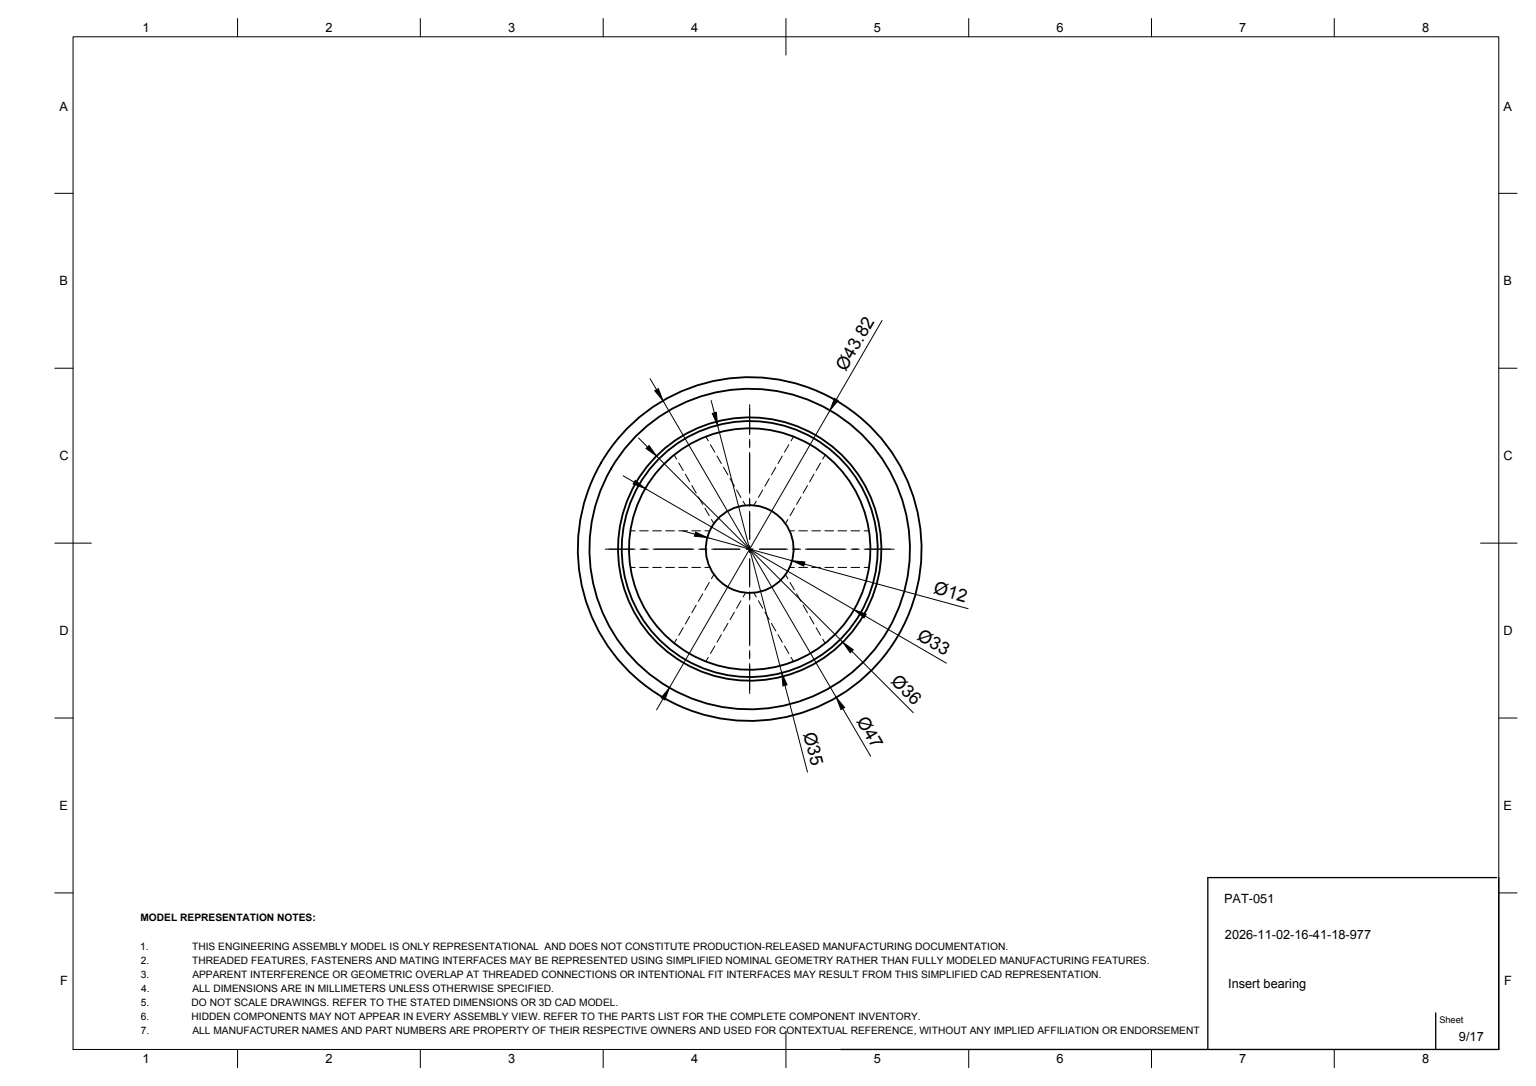
ISO-10303-21;
HEADER;
/* Generated by software containing ST-Developer
 * from STEP Tools, Inc. (www.steptools.com) 
 */

FILE_DESCRIPTION(
/* description */ ('Hand-crank flanged shaft unit'),
/* implementation_level */ '2;1');

FILE_NAME(
/* name */ 'Insert bearing.step',
/* time_stamp */ '2026-10-27T18:35:45-07:00',
/* author */ (''),
/* organization */ (''),
/* preprocessor_version */ 'ST-DEVELOPER v20.2',
/* originating_system */ 'Autodesk Translation Framework v15.17.0.0',
/* authorisation */ '');

FILE_SCHEMA (('AUTOMOTIVE_DESIGN { 1 0 10303 214 3 1 1 }'));
ENDSEC;

DATA;
#10=MECHANICAL_DESIGN_GEOMETRIC_PRESENTATION_REPRESENTATION('',(#289,#290),#6805);
#189=B_SPLINE_CURVE_WITH_KNOTS('',3,(#5317,#5318,#5319,#5320,#5321,#5322,
#5323,#5324,#5325,#5326),.UNSPECIFIED.,.F.,.F.,(4,2,2,2,4),(1.13193471301885,
1.22626174930539,1.32058878559194,1.41491753480854,1.50924628402513),
 .UNSPECIFIED.);
#190=B_SPLINE_CURVE_WITH_KNOTS('',3,(#5328,#5329,#5330,#5331,#5332,#5333,
#5334,#5335,#5336,#5337,#5338,#5339,#5340,#5341,#5342,#5343,#5344,#5345),
 .UNSPECIFIED.,.F.,.F.,(4,2,2,2,2,2,2,2,4),(0.377311571006283,0.471638607292829,
0.565965643579376,0.66029439279597,0.754623142012565,0.84895189122916,0.943280640445754,
1.0376076767323,1.13193471301885),.UNSPECIFIED.);
#191=B_SPLINE_CURVE_WITH_KNOTS('',3,(#5346,#5347,#5348,#5349,#5350,#5351,
#5352,#5353,#5354,#5355),.UNSPECIFIED.,.F.,.F.,(4,2,2,2,4),(1.50924628402513,
1.60357503324173,1.69790378245832,1.79223081874487,1.88655785503141),
 .UNSPECIFIED.);
#192=B_SPLINE_CURVE_WITH_KNOTS('',3,(#5358,#5359,#5360,#5361,#5362,#5363,
#5364,#5365,#5366,#5367,#5368,#5369,#5370,#5371,#5372,#5373,#5374,#5375,
#5376,#5377,#5378,#5379,#5380,#5381,#5382,#5383,#5384,#5385,#5386,#5387,
#5388,#5389,#5390,#5391),.UNSPECIFIED.,.T.,.F.,(4,2,2,2,2,2,2,2,2,2,2,2,
2,2,2,2,4),(0.,0.0955080856649705,0.191016171329941,0.286408845249646,0.38180151916935,
0.477194193089055,0.572586867008759,0.66809495267373,0.763603038338701,
0.859111124003671,0.954619209668642,1.05001188358835,1.14540455750805,1.24079723142776,
1.33618990534746,1.43169799101243,1.5272060766774),.UNSPECIFIED.);
#193=B_SPLINE_CURVE_WITH_KNOTS('',3,(#5394,#5395,#5396,#5397,#5398,#5399,
#5400,#5401,#5402,#5403,#5404,#5405,#5406,#5407,#5408,#5409,#5410,#5411,
#5412,#5413,#5414,#5415,#5416,#5417,#5418,#5419,#5420,#5421,#5422,#5423,
#5424,#5425,#5426,#5427),.UNSPECIFIED.,.T.,.F.,(4,2,2,2,2,2,2,2,2,2,2,2,
2,2,2,2,4),(0.,0.0955080856649706,0.191016171329941,0.286408845249646,0.381801519169351,
0.477194193089055,0.57258686700876,0.668094952673731,0.763603038338701,
0.859111124003672,0.954619209668642,1.05001188358835,1.14540455750805,1.24079723142776,
1.33618990534746,1.43169799101243,1.5272060766774),.UNSPECIFIED.);
#194=B_SPLINE_CURVE_WITH_KNOTS('',3,(#5431,#5432,#5433,#5434,#5435,#5436,
#5437,#5438,#5439,#5440),.UNSPECIFIED.,.F.,.F.,(4,2,2,2,4),(1.13193471301885,
1.22626174930539,1.32058878559194,1.41491753480854,1.50924628402513),
 .UNSPECIFIED.);
#195=B_SPLINE_CURVE_WITH_KNOTS('',3,(#5442,#5443,#5444,#5445,#5446,#5447,
#5448,#5449,#5450,#5451,#5452,#5453,#5454,#5455,#5456,#5457,#5458,#5459),
 .UNSPECIFIED.,.F.,.F.,(4,2,2,2,2,2,2,2,4),(0.377311571006283,0.47163860729283,
0.565965643579376,0.660294392795971,0.754623142012565,0.84895189122916,
0.943280640445755,1.0376076767323,1.13193471301885),.UNSPECIFIED.);
#196=B_SPLINE_CURVE_WITH_KNOTS('',3,(#5460,#5461,#5462,#5463,#5464,#5465,
#5466,#5467,#5468,#5469),.UNSPECIFIED.,.F.,.F.,(4,2,2,2,4),(1.50924628402513,
1.60357503324173,1.69790378245832,1.79223081874487,1.88655785503141),
 .UNSPECIFIED.);
#197=B_SPLINE_CURVE_WITH_KNOTS('',3,(#5478,#5479,#5480,#5481,#5482,#5483,
#5484,#5485,#5486,#5487,#5488,#5489,#5490,#5491,#5492,#5493,#5494,#5495),
 .UNSPECIFIED.,.F.,.F.,(4,2,2,2,2,2,2,2,4),(0.377311571006282,0.471638607292829,
0.565965643579376,0.660294392795971,0.754623142012565,0.84895189122916,
0.943280640445754,1.0376076767323,1.13193471301885),.UNSPECIFIED.);
#198=B_SPLINE_CURVE_WITH_KNOTS('',3,(#5497,#5498,#5499,#5500,#5501,#5502,
#5503,#5504,#5505,#5506),.UNSPECIFIED.,.F.,.F.,(4,2,2,2,4),(1.13193471301885,
1.22626174930539,1.32058878559194,1.41491753480854,1.50924628402513),
 .UNSPECIFIED.);
#199=B_SPLINE_CURVE_WITH_KNOTS('',3,(#5507,#5508,#5509,#5510,#5511,#5512,
#5513,#5514,#5515,#5516),.UNSPECIFIED.,.F.,.F.,(4,2,2,2,4),(1.50924628402513,
1.60357503324172,1.69790378245832,1.79223081874487,1.88655785503141),
 .UNSPECIFIED.);
#200=B_SPLINE_CURVE_WITH_KNOTS('',3,(#5519,#5520,#5521,#5522,#5523,#5524,
#5525,#5526,#5527,#5528,#5529,#5530,#5531,#5532,#5533,#5534,#5535,#5536),
 .UNSPECIFIED.,.F.,.F.,(4,2,2,2,2,2,2,2,4),(0.377311571006283,0.47163860729283,
0.565965643579376,0.660294392795971,0.754623142012565,0.84895189122916,
0.943280640445754,1.0376076767323,1.13193471301885),.UNSPECIFIED.);
#201=B_SPLINE_CURVE_WITH_KNOTS('',3,(#5538,#5539,#5540,#5541,#5542,#5543,
#5544,#5545,#5546,#5547),.UNSPECIFIED.,.F.,.F.,(4,2,2,2,4),(1.13193471301885,
1.22626174930539,1.32058878559194,1.41491753480854,1.50924628402513),
 .UNSPECIFIED.);
#202=B_SPLINE_CURVE_WITH_KNOTS('',3,(#5548,#5549,#5550,#5551,#5552,#5553,
#5554,#5555,#5556,#5557),.UNSPECIFIED.,.F.,.F.,(4,2,2,2,4),(1.50924628402513,
1.60357503324173,1.69790378245832,1.79223081874487,1.88655785503141),
 .UNSPECIFIED.);
#203=B_SPLINE_CURVE_WITH_KNOTS('',3,(#5560,#5561,#5562,#5563,#5564,#5565,
#5566,#5567,#5568,#5569,#5570,#5571,#5572,#5573,#5574,#5575,#5576,#5577),
 .UNSPECIFIED.,.F.,.F.,(4,2,2,2,2,2,2,2,4),(0.377311571006282,0.471638607292829,
0.565965643579376,0.66029439279597,0.754623142012565,0.84895189122916,0.943280640445754,
1.0376076767323,1.13193471301885),.UNSPECIFIED.);
#204=B_SPLINE_CURVE_WITH_KNOTS('',3,(#5579,#5580,#5581,#5582,#5583,#5584,
#5585,#5586,#5587,#5588),.UNSPECIFIED.,.F.,.F.,(4,2,2,2,4),(1.13193471301885,
1.22626174930539,1.32058878559194,1.41491753480854,1.50924628402513),
 .UNSPECIFIED.);
#205=B_SPLINE_CURVE_WITH_KNOTS('',3,(#5589,#5590,#5591,#5592,#5593,#5594,
#5595,#5596,#5597,#5598),.UNSPECIFIED.,.F.,.F.,(4,2,2,2,4),(1.50924628402513,
1.60357503324172,1.69790378245832,1.79223081874487,1.88655785503141),
 .UNSPECIFIED.);
#206=B_SPLINE_CURVE_WITH_KNOTS('',3,(#5601,#5602,#5603,#5604,#5605,#5606,
#5607,#5608,#5609,#5610,#5611,#5612,#5613,#5614,#5615,#5616,#5617,#5618),
 .UNSPECIFIED.,.F.,.F.,(4,2,2,2,2,2,2,2,4),(0.377311571006283,0.471638607292829,
0.565965643579376,0.660294392795971,0.754623142012565,0.84895189122916,
0.943280640445755,1.0376076767323,1.13193471301885),.UNSPECIFIED.);
#207=B_SPLINE_CURVE_WITH_KNOTS('',3,(#5620,#5621,#5622,#5623,#5624,#5625,
#5626,#5627,#5628,#5629),.UNSPECIFIED.,.F.,.F.,(4,2,2,2,4),(1.13193471301885,
1.22626174930539,1.32058878559194,1.41491753480854,1.50924628402513),
 .UNSPECIFIED.);
#208=B_SPLINE_CURVE_WITH_KNOTS('',3,(#5630,#5631,#5632,#5633,#5634,#5635,
#5636,#5637,#5638,#5639),.UNSPECIFIED.,.F.,.F.,(4,2,2,2,4),(1.50924628402513,
1.60357503324172,1.69790378245832,1.79223081874487,1.88655785503141),
 .UNSPECIFIED.);
#209=B_SPLINE_CURVE_WITH_KNOTS('',3,(#5643,#5644,#5645,#5646,#5647,#5648,
#5649,#5650,#5651,#5652,#5653,#5654,#5655,#5656,#5657,#5658,#5659,#5660,
#5661,#5662,#5663,#5664,#5665,#5666,#5667,#5668,#5669,#5670,#5671,#5672,
#5673,#5674,#5675,#5676),.UNSPECIFIED.,.T.,.F.,(4,2,2,2,2,2,2,2,2,2,2,2,
2,2,2,2,4),(0.,0.0955080856649705,0.191016171329941,0.286408845249646,0.38180151916935,
0.477194193089055,0.572586867008759,0.66809495267373,0.7636030383387,0.859111124003671,
0.954619209668642,1.05001188358835,1.14540455750805,1.24079723142776,1.33618990534746,
1.43169799101243,1.5272060766774),.UNSPECIFIED.);
#210=B_SPLINE_CURVE_WITH_KNOTS('',3,(#5679,#5680,#5681,#5682,#5683,#5684,
#5685,#5686,#5687,#5688,#5689,#5690,#5691,#5692,#5693,#5694,#5695,#5696,
#5697,#5698,#5699,#5700,#5701,#5702,#5703,#5704,#5705,#5706,#5707,#5708,
#5709,#5710,#5711,#5712),.UNSPECIFIED.,.T.,.F.,(4,2,2,2,2,2,2,2,2,2,2,2,
2,2,2,2,4),(0.,0.0955080856649706,0.191016171329941,0.286408845249646,0.381801519169351,
0.477194193089055,0.57258686700876,0.668094952673731,0.763603038338701,
0.859111124003672,0.954619209668642,1.05001188358835,1.14540455750805,1.24079723142776,
1.33618990534746,1.43169799101243,1.5272060766774),.UNSPECIFIED.);
#211=B_SPLINE_CURVE_WITH_KNOTS('',3,(#5717,#5718,#5719,#5720,#5721,#5722,
#5723,#5724,#5725,#5726,#5727,#5728,#5729,#5730,#5731,#5732,#5733,#5734,
#5735,#5736,#5737,#5738,#5739,#5740,#5741,#5742,#5743,#5744,#5745,#5746,
#5747,#5748,#5749,#5750),.UNSPECIFIED.,.T.,.F.,(4,2,2,2,2,2,2,2,2,2,2,2,
2,2,2,2,4),(0.,0.0955080856649705,0.191016171329941,0.286408845249646,0.38180151916935,
0.477194193089055,0.572586867008759,0.66809495267373,0.7636030383387,0.859111124003671,
0.954619209668642,1.05001188358835,1.14540455750805,1.24079723142776,1.33618990534746,
1.43169799101243,1.5272060766774),.UNSPECIFIED.);
#212=B_SPLINE_CURVE_WITH_KNOTS('',3,(#5753,#5754,#5755,#5756,#5757,#5758,
#5759,#5760,#5761,#5762,#5763,#5764,#5765,#5766,#5767,#5768,#5769,#5770,
#5771,#5772,#5773,#5774,#5775,#5776,#5777,#5778,#5779,#5780,#5781,#5782,
#5783,#5784,#5785,#5786),.UNSPECIFIED.,.T.,.F.,(4,2,2,2,2,2,2,2,2,2,2,2,
2,2,2,2,4),(0.,0.0955080856649706,0.191016171329941,0.286408845249646,0.381801519169351,
0.477194193089055,0.57258686700876,0.668094952673731,0.763603038338701,
0.859111124003672,0.954619209668642,1.05001188358835,1.14540455750805,1.24079723142776,
1.33618990534746,1.43169799101243,1.5272060766774),.UNSPECIFIED.);
#238=SPHERICAL_SURFACE('',#3719,2.35);
#249=SHAPE_REPRESENTATION_RELATIONSHIP('SRR','None',#6911,#269);
#269=ADVANCED_BREP_SHAPE_REPRESENTATION('',(#310,#311),#6794);
#289=STYLED_ITEM('',(#7091),#310);
#290=STYLED_ITEM('',(#7091),#311);
#310=MANIFOLD_SOLID_BREP('Body1',#3330);
#311=MANIFOLD_SOLID_BREP('Body2',#3331);
#372=FACE_BOUND('',#836,.T.);
#373=FACE_BOUND('',#838,.T.);
#374=FACE_BOUND('',#839,.T.);
#375=FACE_BOUND('',#841,.T.);
#376=FACE_BOUND('',#845,.T.);
#377=FACE_BOUND('',#846,.T.);
#378=FACE_BOUND('',#847,.T.);
#379=FACE_BOUND('',#848,.T.);
#380=FACE_BOUND('',#849,.T.);
#381=FACE_BOUND('',#850,.T.);
#382=FACE_BOUND('',#856,.T.);
#383=FACE_BOUND('',#858,.T.);
#384=FACE_BOUND('',#861,.T.);
#385=FACE_BOUND('',#863,.T.);
#386=FACE_BOUND('',#864,.T.);
#387=FACE_BOUND('',#865,.T.);
#388=FACE_BOUND('',#866,.T.);
#389=FACE_BOUND('',#867,.T.);
#390=FACE_BOUND('',#868,.T.);
#454=PLANE('',#3717);
#455=PLANE('',#3722);
#456=PLANE('',#3732);
#457=PLANE('',#3734);
#458=PLANE('',#3738);
#594=FACE_OUTER_BOUND('',#834,.T.);
#595=FACE_OUTER_BOUND('',#835,.T.);
#596=FACE_OUTER_BOUND('',#837,.T.);
#597=FACE_OUTER_BOUND('',#840,.T.);
#598=FACE_OUTER_BOUND('',#842,.T.);
#599=FACE_OUTER_BOUND('',#843,.T.);
#600=FACE_OUTER_BOUND('',#844,.T.);
#601=FACE_OUTER_BOUND('',#851,.T.);
#602=FACE_OUTER_BOUND('',#852,.T.);
#603=FACE_OUTER_BOUND('',#853,.T.);
#604=FACE_OUTER_BOUND('',#854,.T.);
#605=FACE_OUTER_BOUND('',#855,.T.);
#606=FACE_OUTER_BOUND('',#857,.T.);
#607=FACE_OUTER_BOUND('',#859,.T.);
#608=FACE_OUTER_BOUND('',#860,.T.);
#609=FACE_OUTER_BOUND('',#862,.T.);
#834=EDGE_LOOP('',(#2577,#2578,#2579,#2580));
#835=EDGE_LOOP('',(#2581));
#836=EDGE_LOOP('',(#2582));
#837=EDGE_LOOP('',(#2583,#2584));
#838=EDGE_LOOP('',(#2585));
#839=EDGE_LOOP('',(#2586));
#840=EDGE_LOOP('',(#2587));
#841=EDGE_LOOP('',(#2588));
#842=EDGE_LOOP('',(#2589,#2590,#2591,#2592,#2593,#2594));
#843=EDGE_LOOP('',(#2595,#2596,#2597,#2598,#2599,#2600));
#844=EDGE_LOOP('',(#2601,#2602,#2603,#2604));
#845=EDGE_LOOP('',(#2605,#2606,#2607));
#846=EDGE_LOOP('',(#2608,#2609,#2610));
#847=EDGE_LOOP('',(#2611,#2612,#2613));
#848=EDGE_LOOP('',(#2614,#2615,#2616));
#849=EDGE_LOOP('',(#2617,#2618,#2619));
#850=EDGE_LOOP('',(#2620,#2621,#2622));
#851=EDGE_LOOP('',(#2623,#2624,#2625,#2626,#2627,#2628));
#852=EDGE_LOOP('',(#2629,#2630,#2631,#2632,#2633,#2634));
#853=EDGE_LOOP('',(#2635,#2636,#2637,#2638,#2639,#2640));
#854=EDGE_LOOP('',(#2641,#2642,#2643,#2644,#2645,#2646));
#855=EDGE_LOOP('',(#2647));
#856=EDGE_LOOP('',(#2648));
#857=EDGE_LOOP('',(#2649));
#858=EDGE_LOOP('',(#2650));
#859=EDGE_LOOP('',(#2651,#2652,#2653,#2654));
#860=EDGE_LOOP('',(#2655));
#861=EDGE_LOOP('',(#2656));
#862=EDGE_LOOP('',(#2657,#2658,#2659,#2660));
#863=EDGE_LOOP('',(#2661));
#864=EDGE_LOOP('',(#2662));
#865=EDGE_LOOP('',(#2663));
#866=EDGE_LOOP('',(#2664));
#867=EDGE_LOOP('',(#2665));
#868=EDGE_LOOP('',(#2666));
#1075=LINE('',#5302,#1303);
#1076=LINE('',#5357,#1304);
#1077=LINE('',#5429,#1305);
#1078=LINE('',#5474,#1306);
#1079=LINE('',#5642,#1307);
#1080=LINE('',#5713,#1308);
#1081=LINE('',#5716,#1309);
#1082=LINE('',#5787,#1310);
#1083=LINE('',#5797,#1311);
#1084=LINE('',#5802,#1312);
#1303=VECTOR('',#4358,1.8);
#1304=VECTOR('',#4375,0.25);
#1305=VECTOR('',#4378,0.25);
#1306=VECTOR('',#4383,1.65);
#1307=VECTOR('',#4388,0.25);
#1308=VECTOR('',#4391,0.25);
#1309=VECTOR('',#4394,0.25);
#1310=VECTOR('',#4397,0.25);
#1311=VECTOR('',#4410,1.75);
#1312=VECTOR('',#4417,0.6);
#1506=CIRCLE('',#3715,1.8);
#1507=CIRCLE('',#3716,1.8);
#1508=CIRCLE('',#3718,2.19089023002066);
#1509=CIRCLE('',#3720,2.35);
#1510=CIRCLE('',#3721,2.19089023002066);
#1511=CIRCLE('',#3726,1.65);
#1512=CIRCLE('',#3727,1.65);
#1513=CIRCLE('',#3733,0.6);
#1514=CIRCLE('',#3735,1.75);
#1515=CIRCLE('',#3737,1.75);
#1516=CIRCLE('',#3739,0.6);
#1679=VERTEX_POINT('',#5299);
#1680=VERTEX_POINT('',#5301);
#1681=VERTEX_POINT('',#5305);
#1682=VERTEX_POINT('',#5308);
#1683=VERTEX_POINT('',#5309);
#1684=VERTEX_POINT('',#5311);
#1685=VERTEX_POINT('',#5315);
#1686=VERTEX_POINT('',#5316);
#1687=VERTEX_POINT('',#5327);
#1688=VERTEX_POINT('',#5356);
#1689=VERTEX_POINT('',#5393);
#1690=VERTEX_POINT('',#5428);
#1691=VERTEX_POINT('',#5430);
#1692=VERTEX_POINT('',#5441);
#1693=VERTEX_POINT('',#5471);
#1694=VERTEX_POINT('',#5473);
#1695=VERTEX_POINT('',#5476);
#1696=VERTEX_POINT('',#5477);
#1697=VERTEX_POINT('',#5496);
#1698=VERTEX_POINT('',#5517);
#1699=VERTEX_POINT('',#5518);
#1700=VERTEX_POINT('',#5537);
#1701=VERTEX_POINT('',#5558);
#1702=VERTEX_POINT('',#5559);
#1703=VERTEX_POINT('',#5578);
#1704=VERTEX_POINT('',#5599);
#1705=VERTEX_POINT('',#5600);
#1706=VERTEX_POINT('',#5619);
#1707=VERTEX_POINT('',#5641);
#1708=VERTEX_POINT('',#5678);
#1709=VERTEX_POINT('',#5715);
#1710=VERTEX_POINT('',#5752);
#1711=VERTEX_POINT('',#5789);
#1712=VERTEX_POINT('',#5792);
#1713=VERTEX_POINT('',#5795);
#1714=VERTEX_POINT('',#5799);
#2006=EDGE_CURVE('',#1679,#1679,#1506,.T.);
#2007=EDGE_CURVE('',#1679,#1680,#1075,.T.);
#2008=EDGE_CURVE('',#1680,#1680,#1507,.T.);
#2009=EDGE_CURVE('',#1681,#1681,#1508,.T.);
#2010=EDGE_CURVE('',#1682,#1683,#1509,.T.);
#2011=EDGE_CURVE('',#1684,#1684,#1510,.T.);
#2012=EDGE_CURVE('',#1685,#1686,#189,.T.);
#2013=EDGE_CURVE('',#1687,#1685,#190,.T.);
#2014=EDGE_CURVE('',#1686,#1687,#191,.T.);
#2015=EDGE_CURVE('',#1686,#1688,#1076,.T.);
#2016=EDGE_CURVE('',#1688,#1688,#192,.T.);
#2017=EDGE_CURVE('',#1689,#1689,#193,.T.);
#2018=EDGE_CURVE('',#1689,#1690,#1077,.T.);
#2019=EDGE_CURVE('',#1691,#1690,#194,.T.);
#2020=EDGE_CURVE('',#1692,#1691,#195,.T.);
#2021=EDGE_CURVE('',#1690,#1692,#196,.T.);
#2022=EDGE_CURVE('',#1693,#1693,#1511,.T.);
#2023=EDGE_CURVE('',#1693,#1694,#1078,.T.);
#2024=EDGE_CURVE('',#1694,#1694,#1512,.T.);
#2025=EDGE_CURVE('',#1695,#1696,#197,.T.);
#2026=EDGE_CURVE('',#1696,#1697,#198,.T.);
#2027=EDGE_CURVE('',#1697,#1695,#199,.T.);
#2028=EDGE_CURVE('',#1698,#1699,#200,.T.);
#2029=EDGE_CURVE('',#1699,#1700,#201,.T.);
#2030=EDGE_CURVE('',#1700,#1698,#202,.T.);
#2031=EDGE_CURVE('',#1701,#1702,#203,.T.);
#2032=EDGE_CURVE('',#1702,#1703,#204,.T.);
#2033=EDGE_CURVE('',#1703,#1701,#205,.T.);
#2034=EDGE_CURVE('',#1704,#1705,#206,.T.);
#2035=EDGE_CURVE('',#1705,#1706,#207,.T.);
#2036=EDGE_CURVE('',#1706,#1704,#208,.T.);
#2037=EDGE_CURVE('',#1697,#1707,#1079,.T.);
#2038=EDGE_CURVE('',#1707,#1707,#209,.T.);
#2039=EDGE_CURVE('',#1708,#1708,#210,.T.);
#2040=EDGE_CURVE('',#1708,#1700,#1080,.T.);
#2041=EDGE_CURVE('',#1703,#1709,#1081,.T.);
#2042=EDGE_CURVE('',#1709,#1709,#211,.T.);
#2043=EDGE_CURVE('',#1710,#1710,#212,.T.);
#2044=EDGE_CURVE('',#1710,#1706,#1082,.T.);
#2045=EDGE_CURVE('',#1711,#1711,#1513,.T.);
#2046=EDGE_CURVE('',#1712,#1712,#1514,.T.);
#2047=EDGE_CURVE('',#1713,#1713,#1515,.T.);
#2048=EDGE_CURVE('',#1713,#1712,#1083,.T.);
#2049=EDGE_CURVE('',#1714,#1714,#1516,.T.);
#2050=EDGE_CURVE('',#1714,#1711,#1084,.T.);
#2577=ORIENTED_EDGE('',*,*,#2006,.T.);
#2578=ORIENTED_EDGE('',*,*,#2007,.T.);
#2579=ORIENTED_EDGE('',*,*,#2008,.F.);
#2580=ORIENTED_EDGE('',*,*,#2007,.F.);
#2581=ORIENTED_EDGE('',*,*,#2009,.F.);
#2582=ORIENTED_EDGE('',*,*,#2008,.T.);
#2583=ORIENTED_EDGE('',*,*,#2010,.T.);
#2584=ORIENTED_EDGE('',*,*,#2010,.F.);
#2585=ORIENTED_EDGE('',*,*,#2009,.T.);
#2586=ORIENTED_EDGE('',*,*,#2011,.F.);
#2587=ORIENTED_EDGE('',*,*,#2011,.T.);
#2588=ORIENTED_EDGE('',*,*,#2006,.F.);
#2589=ORIENTED_EDGE('',*,*,#2012,.F.);
#2590=ORIENTED_EDGE('',*,*,#2013,.F.);
#2591=ORIENTED_EDGE('',*,*,#2014,.F.);
#2592=ORIENTED_EDGE('',*,*,#2015,.T.);
#2593=ORIENTED_EDGE('',*,*,#2016,.F.);
#2594=ORIENTED_EDGE('',*,*,#2015,.F.);
#2595=ORIENTED_EDGE('',*,*,#2017,.F.);
#2596=ORIENTED_EDGE('',*,*,#2018,.T.);
#2597=ORIENTED_EDGE('',*,*,#2019,.F.);
#2598=ORIENTED_EDGE('',*,*,#2020,.F.);
#2599=ORIENTED_EDGE('',*,*,#2021,.F.);
#2600=ORIENTED_EDGE('',*,*,#2018,.F.);
#2601=ORIENTED_EDGE('',*,*,#2022,.F.);
#2602=ORIENTED_EDGE('',*,*,#2023,.T.);
#2603=ORIENTED_EDGE('',*,*,#2024,.T.);
#2604=ORIENTED_EDGE('',*,*,#2023,.F.);
#2605=ORIENTED_EDGE('',*,*,#2013,.T.);
#2606=ORIENTED_EDGE('',*,*,#2012,.T.);
#2607=ORIENTED_EDGE('',*,*,#2014,.T.);
#2608=ORIENTED_EDGE('',*,*,#2020,.T.);
#2609=ORIENTED_EDGE('',*,*,#2019,.T.);
#2610=ORIENTED_EDGE('',*,*,#2021,.T.);
#2611=ORIENTED_EDGE('',*,*,#2025,.T.);
#2612=ORIENTED_EDGE('',*,*,#2026,.T.);
#2613=ORIENTED_EDGE('',*,*,#2027,.T.);
#2614=ORIENTED_EDGE('',*,*,#2028,.T.);
#2615=ORIENTED_EDGE('',*,*,#2029,.T.);
#2616=ORIENTED_EDGE('',*,*,#2030,.T.);
#2617=ORIENTED_EDGE('',*,*,#2031,.T.);
#2618=ORIENTED_EDGE('',*,*,#2032,.T.);
#2619=ORIENTED_EDGE('',*,*,#2033,.T.);
#2620=ORIENTED_EDGE('',*,*,#2034,.T.);
#2621=ORIENTED_EDGE('',*,*,#2035,.T.);
#2622=ORIENTED_EDGE('',*,*,#2036,.T.);
#2623=ORIENTED_EDGE('',*,*,#2026,.F.);
#2624=ORIENTED_EDGE('',*,*,#2025,.F.);
#2625=ORIENTED_EDGE('',*,*,#2027,.F.);
#2626=ORIENTED_EDGE('',*,*,#2037,.T.);
#2627=ORIENTED_EDGE('',*,*,#2038,.F.);
#2628=ORIENTED_EDGE('',*,*,#2037,.F.);
#2629=ORIENTED_EDGE('',*,*,#2039,.F.);
#2630=ORIENTED_EDGE('',*,*,#2040,.T.);
#2631=ORIENTED_EDGE('',*,*,#2029,.F.);
#2632=ORIENTED_EDGE('',*,*,#2028,.F.);
#2633=ORIENTED_EDGE('',*,*,#2030,.F.);
#2634=ORIENTED_EDGE('',*,*,#2040,.F.);
#2635=ORIENTED_EDGE('',*,*,#2032,.F.);
#2636=ORIENTED_EDGE('',*,*,#2031,.F.);
#2637=ORIENTED_EDGE('',*,*,#2033,.F.);
#2638=ORIENTED_EDGE('',*,*,#2041,.T.);
#2639=ORIENTED_EDGE('',*,*,#2042,.F.);
#2640=ORIENTED_EDGE('',*,*,#2041,.F.);
#2641=ORIENTED_EDGE('',*,*,#2043,.F.);
#2642=ORIENTED_EDGE('',*,*,#2044,.T.);
#2643=ORIENTED_EDGE('',*,*,#2035,.F.);
#2644=ORIENTED_EDGE('',*,*,#2034,.F.);
#2645=ORIENTED_EDGE('',*,*,#2036,.F.);
#2646=ORIENTED_EDGE('',*,*,#2044,.F.);
#2647=ORIENTED_EDGE('',*,*,#2024,.F.);
#2648=ORIENTED_EDGE('',*,*,#2045,.T.);
#2649=ORIENTED_EDGE('',*,*,#2046,.F.);
#2650=ORIENTED_EDGE('',*,*,#2022,.T.);
#2651=ORIENTED_EDGE('',*,*,#2047,.F.);
#2652=ORIENTED_EDGE('',*,*,#2048,.T.);
#2653=ORIENTED_EDGE('',*,*,#2046,.T.);
#2654=ORIENTED_EDGE('',*,*,#2048,.F.);
#2655=ORIENTED_EDGE('',*,*,#2047,.T.);
#2656=ORIENTED_EDGE('',*,*,#2049,.F.);
#2657=ORIENTED_EDGE('',*,*,#2049,.T.);
#2658=ORIENTED_EDGE('',*,*,#2050,.T.);
#2659=ORIENTED_EDGE('',*,*,#2045,.F.);
#2660=ORIENTED_EDGE('',*,*,#2050,.F.);
#2661=ORIENTED_EDGE('',*,*,#2017,.T.);
#2662=ORIENTED_EDGE('',*,*,#2016,.T.);
#2663=ORIENTED_EDGE('',*,*,#2039,.T.);
#2664=ORIENTED_EDGE('',*,*,#2038,.T.);
#2665=ORIENTED_EDGE('',*,*,#2043,.T.);
#2666=ORIENTED_EDGE('',*,*,#2042,.T.);
#3101=CYLINDRICAL_SURFACE('',#3714,1.8);
#3102=CYLINDRICAL_SURFACE('',#3723,0.25);
#3103=CYLINDRICAL_SURFACE('',#3724,0.25);
#3104=CYLINDRICAL_SURFACE('',#3725,1.65);
#3105=CYLINDRICAL_SURFACE('',#3728,0.25);
#3106=CYLINDRICAL_SURFACE('',#3729,0.25);
#3107=CYLINDRICAL_SURFACE('',#3730,0.25);
#3108=CYLINDRICAL_SURFACE('',#3731,0.25);
#3109=CYLINDRICAL_SURFACE('',#3736,1.75);
#3110=CYLINDRICAL_SURFACE('',#3740,0.6);
#3211=ADVANCED_FACE('',(#594),#3101,.F.);
#3212=ADVANCED_FACE('',(#595,#372),#454,.T.);
#3213=ADVANCED_FACE('',(#596,#373,#374),#238,.T.);
#3214=ADVANCED_FACE('',(#597,#375),#455,.T.);
#3215=ADVANCED_FACE('',(#598),#3102,.F.);
#3216=ADVANCED_FACE('',(#599),#3103,.F.);
#3217=ADVANCED_FACE('',(#600,#376,#377,#378,#379,#380,#381),#3104,.T.);
#3218=ADVANCED_FACE('',(#601),#3105,.F.);
#3219=ADVANCED_FACE('',(#602),#3106,.F.);
#3220=ADVANCED_FACE('',(#603),#3107,.F.);
#3221=ADVANCED_FACE('',(#604),#3108,.F.);
#3222=ADVANCED_FACE('',(#605,#382),#456,.T.);
#3223=ADVANCED_FACE('',(#606,#383),#457,.T.);
#3224=ADVANCED_FACE('',(#607),#3109,.T.);
#3225=ADVANCED_FACE('',(#608,#384),#458,.T.);
#3226=ADVANCED_FACE('',(#609,#385,#386,#387,#388,#389,#390),#3110,.F.);
#3330=CLOSED_SHELL('',(#3211,#3212,#3213,#3214));
#3331=CLOSED_SHELL('',(#3215,#3216,#3217,#3218,#3219,#3220,#3221,#3222,
#3223,#3224,#3225,#3226));
#3713=AXIS2_PLACEMENT_3D('',#5297,#4352,#4353);
#3714=AXIS2_PLACEMENT_3D('',#5298,#4354,#4355);
#3715=AXIS2_PLACEMENT_3D('',#5300,#4356,#4357);
#3716=AXIS2_PLACEMENT_3D('',#5303,#4359,#4360);
#3717=AXIS2_PLACEMENT_3D('',#5304,#4361,#4362);
#3718=AXIS2_PLACEMENT_3D('',#5306,#4363,#4364);
#3719=AXIS2_PLACEMENT_3D('',#5307,#4365,#4366);
#3720=AXIS2_PLACEMENT_3D('',#5310,#4367,#4368);
#3721=AXIS2_PLACEMENT_3D('',#5312,#4369,#4370);
#3722=AXIS2_PLACEMENT_3D('',#5313,#4371,#4372);
#3723=AXIS2_PLACEMENT_3D('',#5314,#4373,#4374);
#3724=AXIS2_PLACEMENT_3D('',#5392,#4376,#4377);
#3725=AXIS2_PLACEMENT_3D('',#5470,#4379,#4380);
#3726=AXIS2_PLACEMENT_3D('',#5472,#4381,#4382);
#3727=AXIS2_PLACEMENT_3D('',#5475,#4384,#4385);
#3728=AXIS2_PLACEMENT_3D('',#5640,#4386,#4387);
#3729=AXIS2_PLACEMENT_3D('',#5677,#4389,#4390);
#3730=AXIS2_PLACEMENT_3D('',#5714,#4392,#4393);
#3731=AXIS2_PLACEMENT_3D('',#5751,#4395,#4396);
#3732=AXIS2_PLACEMENT_3D('',#5788,#4398,#4399);
#3733=AXIS2_PLACEMENT_3D('',#5790,#4400,#4401);
#3734=AXIS2_PLACEMENT_3D('',#5791,#4402,#4403);
#3735=AXIS2_PLACEMENT_3D('',#5793,#4404,#4405);
#3736=AXIS2_PLACEMENT_3D('',#5794,#4406,#4407);
#3737=AXIS2_PLACEMENT_3D('',#5796,#4408,#4409);
#3738=AXIS2_PLACEMENT_3D('',#5798,#4411,#4412);
#3739=AXIS2_PLACEMENT_3D('',#5800,#4413,#4414);
#3740=AXIS2_PLACEMENT_3D('',#5801,#4415,#4416);
#4352=DIRECTION('axis',(0.,0.,1.));
#4353=DIRECTION('refdir',(1.,0.,0.));
#4354=DIRECTION('center_axis',(0.,-1.,0.));
#4355=DIRECTION('ref_axis',(1.,0.,0.));
#4356=DIRECTION('center_axis',(0.,-1.,0.));
#4357=DIRECTION('ref_axis',(1.,0.,0.));
#4358=DIRECTION('',(0.,1.,0.));
#4359=DIRECTION('center_axis',(0.,-1.,0.));
#4360=DIRECTION('ref_axis',(1.,0.,0.));
#4361=DIRECTION('center_axis',(0.,1.,0.));
#4362=DIRECTION('ref_axis',(0.,0.,1.));
#4363=DIRECTION('center_axis',(0.,-1.,0.));
#4364=DIRECTION('ref_axis',(1.,0.,0.));
#4365=DIRECTION('center_axis',(6.12323399573677E-17,0.,1.));
#4366=DIRECTION('ref_axis',(1.,0.,0.));
#4367=DIRECTION('center_axis',(1.22464679914735E-16,-1.,0.));
#4368=DIRECTION('ref_axis',(-1.,-1.22464679914735E-16,0.));
#4369=DIRECTION('center_axis',(0.,-1.,0.));
#4370=DIRECTION('ref_axis',(1.,0.,0.));
#4371=DIRECTION('center_axis',(0.,-1.,0.));
#4372=DIRECTION('ref_axis',(0.,0.,-1.));
#4373=DIRECTION('center_axis',(-0.866025403784438,0.,-0.5));
#4374=DIRECTION('ref_axis',(-0.5,0.,0.866025403784438));
#4375=DIRECTION('',(-0.866025403784438,0.,-0.5));
#4376=DIRECTION('center_axis',(-0.866025403784438,0.,-0.5));
#4377=DIRECTION('ref_axis',(-0.5,0.,0.866025403784438));
#4378=DIRECTION('',(-0.866025403784438,0.,-0.5));
#4379=DIRECTION('center_axis',(0.,-1.,0.));
#4380=DIRECTION('ref_axis',(1.,0.,0.));
#4381=DIRECTION('center_axis',(0.,-1.,0.));
#4382=DIRECTION('ref_axis',(1.,0.,0.));
#4383=DIRECTION('',(0.,1.,0.));
#4384=DIRECTION('center_axis',(0.,-1.,0.));
#4385=DIRECTION('ref_axis',(1.,0.,0.));
#4386=DIRECTION('center_axis',(0.866025403784439,0.,-0.5));
#4387=DIRECTION('ref_axis',(-0.5,0.,-0.866025403784439));
#4388=DIRECTION('',(0.866025403784439,0.,-0.5));
#4389=DIRECTION('center_axis',(0.866025403784439,0.,-0.5));
#4390=DIRECTION('ref_axis',(-0.5,0.,-0.866025403784439));
#4391=DIRECTION('',(0.866025403784439,0.,-0.5));
#4392=DIRECTION('center_axis',(0.,0.,1.));
#4393=DIRECTION('ref_axis',(1.,0.,0.));
#4394=DIRECTION('',(0.,0.,1.));
#4395=DIRECTION('center_axis',(0.,0.,1.));
#4396=DIRECTION('ref_axis',(1.,0.,0.));
#4397=DIRECTION('',(0.,0.,1.));
#4398=DIRECTION('center_axis',(0.,1.,0.));
#4399=DIRECTION('ref_axis',(0.,0.,1.));
#4400=DIRECTION('center_axis',(0.,-1.,0.));
#4401=DIRECTION('ref_axis',(1.,0.,0.));
#4402=DIRECTION('center_axis',(0.,1.,0.));
#4403=DIRECTION('ref_axis',(0.,0.,1.));
#4404=DIRECTION('center_axis',(0.,-1.,0.));
#4405=DIRECTION('ref_axis',(1.,0.,0.));
#4406=DIRECTION('center_axis',(0.,-1.,0.));
#4407=DIRECTION('ref_axis',(1.,0.,0.));
#4408=DIRECTION('center_axis',(0.,-1.,0.));
#4409=DIRECTION('ref_axis',(1.,0.,0.));
#4410=DIRECTION('',(0.,1.,0.));
#4411=DIRECTION('center_axis',(0.,-1.,0.));
#4412=DIRECTION('ref_axis',(0.,0.,-1.));
#4413=DIRECTION('center_axis',(0.,-1.,0.));
#4414=DIRECTION('ref_axis',(1.,0.,0.));
#4415=DIRECTION('center_axis',(0.,-1.,0.));
#4416=DIRECTION('ref_axis',(1.,0.,0.));
#4417=DIRECTION('',(0.,1.,0.));
#5297=CARTESIAN_POINT('',(0.,0.,0.));
#5298=CARTESIAN_POINT('Origin',(0.,0.,0.));
#5299=CARTESIAN_POINT('',(-1.8,-0.85,-2.20436423846524E-16));
#5300=CARTESIAN_POINT('Origin',(0.,-0.85,0.));
#5301=CARTESIAN_POINT('',(-1.8,0.85,-2.20436423846524E-16));
#5302=CARTESIAN_POINT('',(-1.8,0.,-2.20436423846524E-16));
#5303=CARTESIAN_POINT('Origin',(0.,0.85,0.));
#5304=CARTESIAN_POINT('Origin',(2.19089023002066,0.85,0.));
#5305=CARTESIAN_POINT('',(2.19089023002066,0.85,0.));
#5306=CARTESIAN_POINT('Origin',(0.,0.85,0.));
#5307=CARTESIAN_POINT('Origin',(3.99680288865056E-15,0.,0.));
#5308=CARTESIAN_POINT('',(3.85290688975075E-15,-1.76221774462768E-32,2.35));
#5309=CARTESIAN_POINT('',(3.85290688975075E-15,-1.76221774462768E-32,-2.35));
#5310=CARTESIAN_POINT('Origin',(3.99680288865056E-15,0.,0.));
#5311=CARTESIAN_POINT('',(2.19089023002066,-0.85,0.));
#5312=CARTESIAN_POINT('Origin',(0.,-0.85,0.));
#5313=CARTESIAN_POINT('Origin',(1.8,-0.85,0.));
#5314=CARTESIAN_POINT('Origin',(0.,1.55,0.));
#5315=CARTESIAN_POINT('',(1.42894191624432,1.8,0.825000000000001));
#5316=CARTESIAN_POINT('',(1.53744468918255,1.55,0.598968970568896));
#5317=CARTESIAN_POINT('Ctrl Pts',(1.42894191624432,1.8,0.825000000000001));
#5318=CARTESIAN_POINT('Ctrl Pts',(1.44466308895875,1.8,0.797770130104052));
#5319=CARTESIAN_POINT('Ctrl Pts',(1.46055812562105,1.79370633789704,0.768258557763732));
#5320=CARTESIAN_POINT('Ctrl Pts',(1.48824888379079,1.76817777258318,0.713138492740816));
#5321=CARTESIAN_POINT('Ctrl Pts',(1.50008999307766,1.74894552961493,0.687551581002689));
#5322=CARTESIAN_POINT('Ctrl Pts',(1.51812136280714,1.70460745840382,0.646764802471699));
#5323=CARTESIAN_POINT('Ctrl Pts',(1.52552758004446,1.67652816181843,0.628833667319578));
#5324=CARTESIAN_POINT('Ctrl Pts',(1.53516661651472,1.61494799959182,0.604921184808251));
#5325=CARTESIAN_POINT('Ctrl Pts',(1.53744468918255,1.58144291640553,0.598968970568896));
#5326=CARTESIAN_POINT('Ctrl Pts',(1.53744468918255,1.55,0.598968970568896));
#5327=CARTESIAN_POINT('',(1.42894191624432,1.3,0.825000000000001));
#5328=CARTESIAN_POINT('Ctrl Pts',(1.42894191624432,1.3,0.825000000000001));
#5329=CARTESIAN_POINT('Ctrl Pts',(1.4132207435299,1.3,0.852229869895949));
#5330=CARTESIAN_POINT('Ctrl Pts',(1.39561049050871,1.30629366210296,0.880751161609749));
#5331=CARTESIAN_POINT('Ctrl Pts',(1.36172049302549,1.33182222741682,0.932292094146256));
#5332=CARTESIAN_POINT('Ctrl Pts',(1.34548213209931,1.35105447038507,0.955340251466734));
#5333=CARTESIAN_POINT('Ctrl Pts',(1.31917543061769,1.39539254159618,0.99134926498299));
#5334=CARTESIAN_POINT('Ctrl Pts',(1.30734972067592,1.42347183818157,1.00672880483252));
#5335=CARTESIAN_POINT('Ctrl Pts',(1.29146042158868,1.48505200040818,1.02703269653942));
#5336=CARTESIAN_POINT('Ctrl Pts',(1.28744468918255,1.51855708359447,1.03198167246111));
#5337=CARTESIAN_POINT('Ctrl Pts',(1.28744468918255,1.58144291640553,1.03198167246111));
#5338=CARTESIAN_POINT('Ctrl Pts',(1.29146042158868,1.61494799959182,1.02703269653942));
#5339=CARTESIAN_POINT('Ctrl Pts',(1.30734972067592,1.67652816181843,1.00672880483252));
#5340=CARTESIAN_POINT('Ctrl Pts',(1.31917543061769,1.70460745840382,0.991349264982991));
#5341=CARTESIAN_POINT('Ctrl Pts',(1.34548213209931,1.74894552961493,0.955340251466735));
#5342=CARTESIAN_POINT('Ctrl Pts',(1.36172049302549,1.76817777258318,0.932292094146256));
#5343=CARTESIAN_POINT('Ctrl Pts',(1.39561049050871,1.79370633789704,0.880751161609749));
#5344=CARTESIAN_POINT('Ctrl Pts',(1.4132207435299,1.8,0.85222986989595));
#5345=CARTESIAN_POINT('Ctrl Pts',(1.42894191624432,1.8,0.825000000000001));
#5346=CARTESIAN_POINT('Ctrl Pts',(1.53744468918255,1.55,0.598968970568896));
#5347=CARTESIAN_POINT('Ctrl Pts',(1.53744468918255,1.51855708359447,0.598968970568896));
#5348=CARTESIAN_POINT('Ctrl Pts',(1.53516661651472,1.48505200040818,0.60492118480825));
#5349=CARTESIAN_POINT('Ctrl Pts',(1.52552758004446,1.42347183818157,0.628833667319578));
#5350=CARTESIAN_POINT('Ctrl Pts',(1.51812136280714,1.39539254159618,0.646764802471699));
#5351=CARTESIAN_POINT('Ctrl Pts',(1.50008999307766,1.35105447038507,0.687551581002689));
#5352=CARTESIAN_POINT('Ctrl Pts',(1.48824888379079,1.33182222741682,0.713138492740816));
#5353=CARTESIAN_POINT('Ctrl Pts',(1.46055812562105,1.30629366210296,0.768258557763732));
#5354=CARTESIAN_POINT('Ctrl Pts',(1.44466308895875,1.3,0.797770130104052));
#5355=CARTESIAN_POINT('Ctrl Pts',(1.42894191624432,1.3,0.825000000000001));
#5356=CARTESIAN_POINT('',(0.59736109069228,1.55,0.0562114519197835));
#5357=CARTESIAN_POINT('',(0.125,1.55,-0.21650635094611));
#5358=CARTESIAN_POINT('Ctrl Pts',(0.59736109069228,1.55,0.0562114519197835));
#5359=CARTESIAN_POINT('Ctrl Pts',(0.59736109069228,1.58183602855499,0.0562114519197835));
#5360=CARTESIAN_POINT('Ctrl Pts',(0.596809586309859,1.61548166177648,0.0633319361811907));
#5361=CARTESIAN_POINT('Ctrl Pts',(0.593243052195919,1.67693412158597,0.0908585874761106));
#5362=CARTESIAN_POINT('Ctrl Pts',(0.590063593315144,1.70478184753241,0.111151766652641));
#5363=CARTESIAN_POINT('Ctrl Pts',(0.579820497891285,1.74874496453875,0.15600214762839));
#5364=CARTESIAN_POINT('Ctrl Pts',(0.572042315803119,1.76792916820474,0.183678633836535));
#5365=CARTESIAN_POINT('Ctrl Pts',(0.549947124580676,1.79356669468566,0.241926459727039));
#5366=CARTESIAN_POINT('Ctrl Pts',(0.53551402125728,1.8,0.27246250701687));
#5367=CARTESIAN_POINT('Ctrl Pts',(0.503716463284046,1.8,0.32753749298313));
#5368=CARTESIAN_POINT('Ctrl Pts',(0.484488022261586,1.79356669468566,0.355304950761552));
#5369=CARTESIAN_POINT('Ctrl Pts',(0.445091520936419,1.76792916820474,0.403563860606914));
#5370=CARTESIAN_POINT('Ctrl Pts',(0.425012071836758,1.74874496453875,0.4241382069946));
#5371=CARTESIAN_POINT('Ctrl Pts',(0.391292050254278,1.70478184753241,0.455434178332924));
#5372=CARTESIAN_POINT('Ctrl Pts',(0.375307371004241,1.67693412158597,0.468334260082228));
#5373=CARTESIAN_POINT('Ctrl Pts',(0.353251858758695,1.61548166177647,0.485186294875824));
#5374=CARTESIAN_POINT('Ctrl Pts',(0.347361090692279,1.58183602855499,0.489224153812003));
#5375=CARTESIAN_POINT('Ctrl Pts',(0.347361090692279,1.51816397144501,0.489224153812003));
#5376=CARTESIAN_POINT('Ctrl Pts',(0.353251858758695,1.48451833822352,0.485186294875824));
#5377=CARTESIAN_POINT('Ctrl Pts',(0.375307371004241,1.42306587841403,0.468334260082228));
#5378=CARTESIAN_POINT('Ctrl Pts',(0.391292050254278,1.39521815246759,0.455434178332924));
#5379=CARTESIAN_POINT('Ctrl Pts',(0.425012071836758,1.35125503546125,0.4241382069946));
#5380=CARTESIAN_POINT('Ctrl Pts',(0.445091520936418,1.33207083179526,0.403563860606914));
#5381=CARTESIAN_POINT('Ctrl Pts',(0.484488022261586,1.30643330531434,0.355304950761552));
#5382=CARTESIAN_POINT('Ctrl Pts',(0.503716463284046,1.3,0.32753749298313));
#5383=CARTESIAN_POINT('Ctrl Pts',(0.53551402125728,1.3,0.27246250701687));
#5384=CARTESIAN_POINT('Ctrl Pts',(0.549947124580676,1.30643330531434,0.241926459727039));
#5385=CARTESIAN_POINT('Ctrl Pts',(0.572042315803119,1.33207083179526,0.183678633836535));
#5386=CARTESIAN_POINT('Ctrl Pts',(0.579820497891285,1.35125503546125,0.15600214762839));
#5387=CARTESIAN_POINT('Ctrl Pts',(0.590063593315144,1.39521815246759,0.111151766652641));
#5388=CARTESIAN_POINT('Ctrl Pts',(0.593243052195919,1.42306587841403,0.0908585874761105));
#5389=CARTESIAN_POINT('Ctrl Pts',(0.596809586309859,1.48451833822352,0.0633319361811906));
#5390=CARTESIAN_POINT('Ctrl Pts',(0.59736109069228,1.51816397144501,0.0562114519197835));
#5391=CARTESIAN_POINT('Ctrl Pts',(0.59736109069228,1.55,0.0562114519197835));
#5392=CARTESIAN_POINT('Origin',(0.,1.55,0.));
#5393=CARTESIAN_POINT('',(-0.347361090692279,1.55,-0.489224153812003));
#5394=CARTESIAN_POINT('Ctrl Pts',(-0.347361090692279,1.55,-0.489224153812003));
#5395=CARTESIAN_POINT('Ctrl Pts',(-0.347361090692279,1.51816397144501,-0.489224153812003));
#5396=CARTESIAN_POINT('Ctrl Pts',(-0.353251858758695,1.48451833822352,-0.485186294875824));
#5397=CARTESIAN_POINT('Ctrl Pts',(-0.375307371004241,1.42306587841403,-0.468334260082228));
#5398=CARTESIAN_POINT('Ctrl Pts',(-0.391292050254278,1.39521815246759,-0.455434178332924));
#5399=CARTESIAN_POINT('Ctrl Pts',(-0.425012071836758,1.35125503546125,-0.4241382069946));
#5400=CARTESIAN_POINT('Ctrl Pts',(-0.445091520936419,1.33207083179526,-0.403563860606914));
#5401=CARTESIAN_POINT('Ctrl Pts',(-0.484488022261586,1.30643330531434,-0.355304950761552));
#5402=CARTESIAN_POINT('Ctrl Pts',(-0.503716463284046,1.3,-0.32753749298313));
#5403=CARTESIAN_POINT('Ctrl Pts',(-0.53551402125728,1.3,-0.27246250701687));
#5404=CARTESIAN_POINT('Ctrl Pts',(-0.549947124580676,1.30643330531434,-0.241926459727039));
#5405=CARTESIAN_POINT('Ctrl Pts',(-0.572042315803119,1.33207083179526,-0.183678633836535));
#5406=CARTESIAN_POINT('Ctrl Pts',(-0.579820497891285,1.35125503546125,-0.15600214762839));
#5407=CARTESIAN_POINT('Ctrl Pts',(-0.590063593315144,1.39521815246759,-0.111151766652641));
#5408=CARTESIAN_POINT('Ctrl Pts',(-0.593243052195918,1.42306587841403,-0.0908585874761106));
#5409=CARTESIAN_POINT('Ctrl Pts',(-0.596809586309859,1.48451833822352,-0.0633319361811906));
#5410=CARTESIAN_POINT('Ctrl Pts',(-0.597361090692279,1.51816397144501,-0.0562114519197835));
#5411=CARTESIAN_POINT('Ctrl Pts',(-0.597361090692279,1.58183602855499,-0.0562114519197835));
#5412=CARTESIAN_POINT('Ctrl Pts',(-0.596809586309859,1.61548166177647,-0.0633319361811905));
#5413=CARTESIAN_POINT('Ctrl Pts',(-0.593243052195918,1.67693412158597,-0.0908585874761104));
#5414=CARTESIAN_POINT('Ctrl Pts',(-0.590063593315144,1.70478184753241,-0.111151766652641));
#5415=CARTESIAN_POINT('Ctrl Pts',(-0.579820497891285,1.74874496453875,-0.15600214762839));
#5416=CARTESIAN_POINT('Ctrl Pts',(-0.572042315803118,1.76792916820474,-0.183678633836535));
#5417=CARTESIAN_POINT('Ctrl Pts',(-0.549947124580676,1.79356669468566,-0.241926459727039));
#5418=CARTESIAN_POINT('Ctrl Pts',(-0.53551402125728,1.8,-0.27246250701687));
#5419=CARTESIAN_POINT('Ctrl Pts',(-0.503716463284046,1.8,-0.32753749298313));
#5420=CARTESIAN_POINT('Ctrl Pts',(-0.484488022261586,1.79356669468566,-0.355304950761552));
#5421=CARTESIAN_POINT('Ctrl Pts',(-0.445091520936419,1.76792916820474,-0.403563860606914));
#5422=CARTESIAN_POINT('Ctrl Pts',(-0.425012071836758,1.74874496453875,-0.4241382069946));
#5423=CARTESIAN_POINT('Ctrl Pts',(-0.391292050254278,1.70478184753241,-0.455434178332924));
#5424=CARTESIAN_POINT('Ctrl Pts',(-0.375307371004241,1.67693412158597,-0.468334260082228));
#5425=CARTESIAN_POINT('Ctrl Pts',(-0.353251858758695,1.61548166177648,-0.485186294875824));
#5426=CARTESIAN_POINT('Ctrl Pts',(-0.347361090692279,1.58183602855499,-0.489224153812003));
#5427=CARTESIAN_POINT('Ctrl Pts',(-0.347361090692279,1.55,-0.489224153812003));
#5428=CARTESIAN_POINT('',(-1.28744468918255,1.55,-1.03198167246111));
#5429=CARTESIAN_POINT('',(0.125,1.55,-0.21650635094611));
#5430=CARTESIAN_POINT('',(-1.42894191624432,1.3,-0.825000000000001));
#5431=CARTESIAN_POINT('Ctrl Pts',(-1.42894191624432,1.3,-0.825000000000001));
#5432=CARTESIAN_POINT('Ctrl Pts',(-1.4132207435299,1.3,-0.852229869895949));
#5433=CARTESIAN_POINT('Ctrl Pts',(-1.39561049050871,1.30629366210296,-0.880751161609749));
#5434=CARTESIAN_POINT('Ctrl Pts',(-1.36172049302549,1.33182222741682,-0.932292094146256));
#5435=CARTESIAN_POINT('Ctrl Pts',(-1.34548213209931,1.35105447038507,-0.955340251466735));
#5436=CARTESIAN_POINT('Ctrl Pts',(-1.31917543061769,1.39539254159618,-0.991349264982991));
#5437=CARTESIAN_POINT('Ctrl Pts',(-1.30734972067592,1.42347183818157,-1.00672880483252));
#5438=CARTESIAN_POINT('Ctrl Pts',(-1.29146042158868,1.48505200040818,-1.02703269653942));
#5439=CARTESIAN_POINT('Ctrl Pts',(-1.28744468918255,1.51855708359447,-1.03198167246111));
#5440=CARTESIAN_POINT('Ctrl Pts',(-1.28744468918255,1.55,-1.03198167246111));
#5441=CARTESIAN_POINT('',(-1.42894191624432,1.8,-0.825000000000001));
#5442=CARTESIAN_POINT('Ctrl Pts',(-1.42894191624432,1.8,-0.825000000000001));
#5443=CARTESIAN_POINT('Ctrl Pts',(-1.44466308895875,1.8,-0.797770130104052));
#5444=CARTESIAN_POINT('Ctrl Pts',(-1.46055812562105,1.79370633789704,-0.768258557763732));
#5445=CARTESIAN_POINT('Ctrl Pts',(-1.48824888379079,1.76817777258318,-0.713138492740816));
#5446=CARTESIAN_POINT('Ctrl Pts',(-1.50008999307766,1.74894552961493,-0.687551581002689));
#5447=CARTESIAN_POINT('Ctrl Pts',(-1.51812136280714,1.70460745840382,-0.646764802471699));
#5448=CARTESIAN_POINT('Ctrl Pts',(-1.52552758004446,1.67652816181843,-0.628833667319578));
#5449=CARTESIAN_POINT('Ctrl Pts',(-1.53516661651472,1.61494799959182,-0.60492118480825));
#5450=CARTESIAN_POINT('Ctrl Pts',(-1.53744468918255,1.58144291640553,-0.598968970568896));
#5451=CARTESIAN_POINT('Ctrl Pts',(-1.53744468918255,1.51855708359447,-0.598968970568896));
#5452=CARTESIAN_POINT('Ctrl Pts',(-1.53516661651472,1.48505200040818,-0.60492118480825));
#5453=CARTESIAN_POINT('Ctrl Pts',(-1.52552758004446,1.42347183818157,-0.628833667319578));
#5454=CARTESIAN_POINT('Ctrl Pts',(-1.51812136280714,1.39539254159618,-0.646764802471699));
#5455=CARTESIAN_POINT('Ctrl Pts',(-1.50008999307766,1.35105447038507,-0.687551581002689));
#5456=CARTESIAN_POINT('Ctrl Pts',(-1.48824888379079,1.33182222741682,-0.713138492740816));
#5457=CARTESIAN_POINT('Ctrl Pts',(-1.46055812562105,1.30629366210296,-0.768258557763732));
#5458=CARTESIAN_POINT('Ctrl Pts',(-1.44466308895875,1.3,-0.797770130104052));
#5459=CARTESIAN_POINT('Ctrl Pts',(-1.42894191624432,1.3,-0.825000000000001));
#5460=CARTESIAN_POINT('Ctrl Pts',(-1.28744468918255,1.55,-1.03198167246111));
#5461=CARTESIAN_POINT('Ctrl Pts',(-1.28744468918255,1.58144291640553,-1.03198167246111));
#5462=CARTESIAN_POINT('Ctrl Pts',(-1.29146042158868,1.61494799959182,-1.02703269653942));
#5463=CARTESIAN_POINT('Ctrl Pts',(-1.30734972067592,1.67652816181843,-1.00672880483252));
#5464=CARTESIAN_POINT('Ctrl Pts',(-1.31917543061769,1.70460745840382,-0.991349264982991));
#5465=CARTESIAN_POINT('Ctrl Pts',(-1.34548213209931,1.74894552961493,-0.955340251466734));
#5466=CARTESIAN_POINT('Ctrl Pts',(-1.36172049302549,1.76817777258318,-0.932292094146256));
#5467=CARTESIAN_POINT('Ctrl Pts',(-1.39561049050871,1.79370633789704,-0.880751161609749));
#5468=CARTESIAN_POINT('Ctrl Pts',(-1.4132207435299,1.8,-0.852229869895949));
#5469=CARTESIAN_POINT('Ctrl Pts',(-1.42894191624432,1.8,-0.825000000000001));
#5470=CARTESIAN_POINT('Origin',(0.,1.55,0.));
#5471=CARTESIAN_POINT('',(-1.65,0.85,-2.02066721859313E-16));
#5472=CARTESIAN_POINT('Origin',(0.,0.85,0.));
#5473=CARTESIAN_POINT('',(-1.65,2.25,-2.02066721859313E-16));
#5474=CARTESIAN_POINT('',(-1.65,1.55,-2.02066721859313E-16));
#5475=CARTESIAN_POINT('Origin',(0.,2.25,0.));
#5476=CARTESIAN_POINT('',(-1.42894191624432,1.3,0.825));
#5477=CARTESIAN_POINT('',(-1.42894191624432,1.8,0.825));
#5478=CARTESIAN_POINT('Ctrl Pts',(-1.42894191624432,1.3,0.825));
#5479=CARTESIAN_POINT('Ctrl Pts',(-1.44466308895875,1.3,0.797770130104051));
#5480=CARTESIAN_POINT('Ctrl Pts',(-1.46055812562105,1.30629366210296,0.768258557763731));
#5481=CARTESIAN_POINT('Ctrl Pts',(-1.48824888379079,1.33182222741682,0.713138492740815));
#5482=CARTESIAN_POINT('Ctrl Pts',(-1.50008999307766,1.35105447038507,0.687551581002688));
#5483=CARTESIAN_POINT('Ctrl Pts',(-1.51812136280714,1.39539254159618,0.646764802471698));
#5484=CARTESIAN_POINT('Ctrl Pts',(-1.52552758004446,1.42347183818157,0.628833667319577));
#5485=CARTESIAN_POINT('Ctrl Pts',(-1.53516661651472,1.48505200040818,0.604921184808249));
#5486=CARTESIAN_POINT('Ctrl Pts',(-1.53744468918255,1.51855708359447,0.598968970568895));
#5487=CARTESIAN_POINT('Ctrl Pts',(-1.53744468918255,1.58144291640553,0.598968970568895));
#5488=CARTESIAN_POINT('Ctrl Pts',(-1.53516661651472,1.61494799959182,0.604921184808249));
#5489=CARTESIAN_POINT('Ctrl Pts',(-1.52552758004446,1.67652816181843,0.628833667319577));
#5490=CARTESIAN_POINT('Ctrl Pts',(-1.51812136280714,1.70460745840382,0.646764802471698));
#5491=CARTESIAN_POINT('Ctrl Pts',(-1.50008999307766,1.74894552961493,0.687551581002688));
#5492=CARTESIAN_POINT('Ctrl Pts',(-1.48824888379079,1.76817777258318,0.713138492740815));
#5493=CARTESIAN_POINT('Ctrl Pts',(-1.46055812562105,1.79370633789704,0.768258557763731));
#5494=CARTESIAN_POINT('Ctrl Pts',(-1.44466308895875,1.8,0.797770130104051));
#5495=CARTESIAN_POINT('Ctrl Pts',(-1.42894191624432,1.8,0.825));
#5496=CARTESIAN_POINT('',(-1.28744468918255,1.55,1.03198167246111));
#5497=CARTESIAN_POINT('Ctrl Pts',(-1.42894191624432,1.8,0.825));
#5498=CARTESIAN_POINT('Ctrl Pts',(-1.4132207435299,1.8,0.852229869895948));
#5499=CARTESIAN_POINT('Ctrl Pts',(-1.39561049050871,1.79370633789704,0.880751161609747));
#5500=CARTESIAN_POINT('Ctrl Pts',(-1.36172049302549,1.76817777258318,0.932292094146255));
#5501=CARTESIAN_POINT('Ctrl Pts',(-1.34548213209931,1.74894552961493,0.955340251466733));
#5502=CARTESIAN_POINT('Ctrl Pts',(-1.31917543061769,1.70460745840382,0.991349264982989));
#5503=CARTESIAN_POINT('Ctrl Pts',(-1.30734972067592,1.67652816181843,1.00672880483252));
#5504=CARTESIAN_POINT('Ctrl Pts',(-1.29146042158868,1.61494799959182,1.02703269653942));
#5505=CARTESIAN_POINT('Ctrl Pts',(-1.28744468918255,1.58144291640553,1.03198167246111));
#5506=CARTESIAN_POINT('Ctrl Pts',(-1.28744468918255,1.55,1.03198167246111));
#5507=CARTESIAN_POINT('Ctrl Pts',(-1.28744468918255,1.55,1.03198167246111));
#5508=CARTESIAN_POINT('Ctrl Pts',(-1.28744468918255,1.51855708359447,1.03198167246111));
#5509=CARTESIAN_POINT('Ctrl Pts',(-1.29146042158868,1.48505200040818,1.02703269653942));
#5510=CARTESIAN_POINT('Ctrl Pts',(-1.30734972067592,1.42347183818157,1.00672880483252));
#5511=CARTESIAN_POINT('Ctrl Pts',(-1.31917543061769,1.39539254159618,0.99134926498299));
#5512=CARTESIAN_POINT('Ctrl Pts',(-1.34548213209931,1.35105447038508,0.955340251466733));
#5513=CARTESIAN_POINT('Ctrl Pts',(-1.36172049302549,1.33182222741682,0.932292094146255));
#5514=CARTESIAN_POINT('Ctrl Pts',(-1.39561049050871,1.30629366210296,0.880751161609748));
#5515=CARTESIAN_POINT('Ctrl Pts',(-1.4132207435299,1.3,0.852229869895949));
#5516=CARTESIAN_POINT('Ctrl Pts',(-1.42894191624432,1.3,0.825));
#5517=CARTESIAN_POINT('',(1.42894191624432,1.8,-0.825));
#5518=CARTESIAN_POINT('',(1.42894191624432,1.3,-0.825));
#5519=CARTESIAN_POINT('Ctrl Pts',(1.42894191624432,1.8,-0.825));
#5520=CARTESIAN_POINT('Ctrl Pts',(1.4132207435299,1.8,-0.852229869895949));
#5521=CARTESIAN_POINT('Ctrl Pts',(1.39561049050871,1.79370633789704,-0.880751161609748));
#5522=CARTESIAN_POINT('Ctrl Pts',(1.36172049302549,1.76817777258318,-0.932292094146255));
#5523=CARTESIAN_POINT('Ctrl Pts',(1.34548213209931,1.74894552961493,-0.955340251466734));
#5524=CARTESIAN_POINT('Ctrl Pts',(1.31917543061769,1.70460745840382,-0.99134926498299));
#5525=CARTESIAN_POINT('Ctrl Pts',(1.30734972067592,1.67652816181843,-1.00672880483252));
#5526=CARTESIAN_POINT('Ctrl Pts',(1.29146042158868,1.61494799959182,-1.02703269653942));
#5527=CARTESIAN_POINT('Ctrl Pts',(1.28744468918255,1.58144291640553,-1.03198167246111));
#5528=CARTESIAN_POINT('Ctrl Pts',(1.28744468918255,1.51855708359447,-1.03198167246111));
#5529=CARTESIAN_POINT('Ctrl Pts',(1.29146042158868,1.48505200040818,-1.02703269653942));
#5530=CARTESIAN_POINT('Ctrl Pts',(1.30734972067592,1.42347183818157,-1.00672880483252));
#5531=CARTESIAN_POINT('Ctrl Pts',(1.31917543061769,1.39539254159618,-0.99134926498299));
#5532=CARTESIAN_POINT('Ctrl Pts',(1.34548213209931,1.35105447038507,-0.955340251466734));
#5533=CARTESIAN_POINT('Ctrl Pts',(1.36172049302549,1.33182222741682,-0.932292094146255));
#5534=CARTESIAN_POINT('Ctrl Pts',(1.39561049050871,1.30629366210296,-0.880751161609748));
#5535=CARTESIAN_POINT('Ctrl Pts',(1.4132207435299,1.3,-0.852229869895948));
#5536=CARTESIAN_POINT('Ctrl Pts',(1.42894191624432,1.3,-0.825));
#5537=CARTESIAN_POINT('',(1.53744468918255,1.55,-0.598968970568895));
#5538=CARTESIAN_POINT('Ctrl Pts',(1.42894191624432,1.3,-0.825));
#5539=CARTESIAN_POINT('Ctrl Pts',(1.44466308895875,1.3,-0.797770130104051));
#5540=CARTESIAN_POINT('Ctrl Pts',(1.46055812562105,1.30629366210296,-0.768258557763731));
#5541=CARTESIAN_POINT('Ctrl Pts',(1.48824888379079,1.33182222741682,-0.713138492740815));
#5542=CARTESIAN_POINT('Ctrl Pts',(1.50008999307766,1.35105447038507,-0.687551581002688));
#5543=CARTESIAN_POINT('Ctrl Pts',(1.51812136280714,1.39539254159618,-0.646764802471698));
#5544=CARTESIAN_POINT('Ctrl Pts',(1.52552758004446,1.42347183818157,-0.628833667319577));
#5545=CARTESIAN_POINT('Ctrl Pts',(1.53516661651472,1.48505200040818,-0.604921184808249));
#5546=CARTESIAN_POINT('Ctrl Pts',(1.53744468918255,1.51855708359447,-0.598968970568895));
#5547=CARTESIAN_POINT('Ctrl Pts',(1.53744468918255,1.55,-0.598968970568895));
#5548=CARTESIAN_POINT('Ctrl Pts',(1.53744468918255,1.55,-0.598968970568895));
#5549=CARTESIAN_POINT('Ctrl Pts',(1.53744468918255,1.58144291640553,-0.598968970568895));
#5550=CARTESIAN_POINT('Ctrl Pts',(1.53516661651472,1.61494799959182,-0.604921184808249));
#5551=CARTESIAN_POINT('Ctrl Pts',(1.52552758004446,1.67652816181843,-0.628833667319577));
#5552=CARTESIAN_POINT('Ctrl Pts',(1.51812136280714,1.70460745840382,-0.646764802471698));
#5553=CARTESIAN_POINT('Ctrl Pts',(1.50008999307766,1.74894552961493,-0.687551581002688));
#5554=CARTESIAN_POINT('Ctrl Pts',(1.48824888379079,1.76817777258318,-0.713138492740815));
#5555=CARTESIAN_POINT('Ctrl Pts',(1.46055812562105,1.79370633789704,-0.768258557763731));
#5556=CARTESIAN_POINT('Ctrl Pts',(1.44466308895875,1.8,-0.797770130104051));
#5557=CARTESIAN_POINT('Ctrl Pts',(1.42894191624432,1.8,-0.825));
#5558=CARTESIAN_POINT('',(0.,1.3,-1.65));
#5559=CARTESIAN_POINT('',(0.,1.8,-1.65));
#5560=CARTESIAN_POINT('Ctrl Pts',(1.38777878078145E-17,1.3,-1.65));
#5561=CARTESIAN_POINT('Ctrl Pts',(0.0314423454288489,1.3,-1.65));
#5562=CARTESIAN_POINT('Ctrl Pts',(0.0649476351123396,1.30629366210296,-1.64900971937348));
#5563=CARTESIAN_POINT('Ctrl Pts',(0.126528390765307,1.33182222741682,-1.64543058688707));
#5564=CARTESIAN_POINT('Ctrl Pts',(0.154607860978348,1.35105447038507,-1.64289183246942));
#5565=CARTESIAN_POINT('Ctrl Pts',(0.198945932189457,1.39539254159618,-1.63811406745469));
#5566=CARTESIAN_POINT('Ctrl Pts',(0.218177859368546,1.42347183818157,-1.63556247215209));
#5567=CARTESIAN_POINT('Ctrl Pts',(0.243706194926033,1.48505200040818,-1.63195388134767));
#5568=CARTESIAN_POINT('Ctrl Pts',(0.25,1.51855708359447,-1.63095064303001));
#5569=CARTESIAN_POINT('Ctrl Pts',(0.25,1.58144291640553,-1.63095064303001));
#5570=CARTESIAN_POINT('Ctrl Pts',(0.243706194926033,1.61494799959182,-1.63195388134767));
#5571=CARTESIAN_POINT('Ctrl Pts',(0.218177859368546,1.67652816181843,-1.63556247215209));
#5572=CARTESIAN_POINT('Ctrl Pts',(0.198945932189457,1.70460745840382,-1.63811406745469));
#5573=CARTESIAN_POINT('Ctrl Pts',(0.154607860978349,1.74894552961493,-1.64289183246942));
#5574=CARTESIAN_POINT('Ctrl Pts',(0.126528390765307,1.76817777258318,-1.64543058688707));
#5575=CARTESIAN_POINT('Ctrl Pts',(0.0649476351123398,1.79370633789704,-1.64900971937348));
#5576=CARTESIAN_POINT('Ctrl Pts',(0.031442345428849,1.8,-1.65));
#5577=CARTESIAN_POINT('Ctrl Pts',(7.63278329429795E-17,1.8,-1.65));
#5578=CARTESIAN_POINT('',(-0.25,1.55,-1.63095064303001));
#5579=CARTESIAN_POINT('Ctrl Pts',(9.0205620750794E-17,1.8,-1.65));
#5580=CARTESIAN_POINT('Ctrl Pts',(-0.0314423454288488,1.8,-1.65));
#5581=CARTESIAN_POINT('Ctrl Pts',(-0.0649476351123396,1.79370633789704,
-1.64900971937348));
#5582=CARTESIAN_POINT('Ctrl Pts',(-0.126528390765307,1.76817777258318,-1.64543058688707));
#5583=CARTESIAN_POINT('Ctrl Pts',(-0.154607860978348,1.74894552961493,-1.64289183246942));
#5584=CARTESIAN_POINT('Ctrl Pts',(-0.198945932189456,1.70460745840382,-1.63811406745469));
#5585=CARTESIAN_POINT('Ctrl Pts',(-0.218177859368546,1.67652816181843,-1.63556247215209));
#5586=CARTESIAN_POINT('Ctrl Pts',(-0.243706194926033,1.61494799959182,-1.63195388134767));
#5587=CARTESIAN_POINT('Ctrl Pts',(-0.25,1.58144291640553,-1.63095064303001));
#5588=CARTESIAN_POINT('Ctrl Pts',(-0.25,1.55,-1.63095064303001));
#5589=CARTESIAN_POINT('Ctrl Pts',(-0.25,1.55,-1.63095064303001));
#5590=CARTESIAN_POINT('Ctrl Pts',(-0.25,1.51855708359447,-1.63095064303001));
#5591=CARTESIAN_POINT('Ctrl Pts',(-0.243706194926033,1.48505200040818,-1.63195388134767));
#5592=CARTESIAN_POINT('Ctrl Pts',(-0.218177859368546,1.42347183818157,-1.63556247215209));
#5593=CARTESIAN_POINT('Ctrl Pts',(-0.198945932189457,1.39539254159618,-1.63811406745469));
#5594=CARTESIAN_POINT('Ctrl Pts',(-0.154607860978349,1.35105447038507,-1.64289183246942));
#5595=CARTESIAN_POINT('Ctrl Pts',(-0.126528390765307,1.33182222741682,-1.64543058688707));
#5596=CARTESIAN_POINT('Ctrl Pts',(-0.0649476351123398,1.30629366210296,
-1.64900971937348));
#5597=CARTESIAN_POINT('Ctrl Pts',(-0.031442345428849,1.3,-1.65));
#5598=CARTESIAN_POINT('Ctrl Pts',(-4.85722573273506E-17,1.3,-1.65));
#5599=CARTESIAN_POINT('',(0.,1.8,1.65));
#5600=CARTESIAN_POINT('',(0.,1.3,1.65));
#5601=CARTESIAN_POINT('Ctrl Pts',(8.32667268468867E-17,1.8,1.65));
#5602=CARTESIAN_POINT('Ctrl Pts',(0.031442345428849,1.8,1.65));
#5603=CARTESIAN_POINT('Ctrl Pts',(0.0649476351123398,1.79370633789704,1.64900971937348));
#5604=CARTESIAN_POINT('Ctrl Pts',(0.126528390765307,1.76817777258318,1.64543058688707));
#5605=CARTESIAN_POINT('Ctrl Pts',(0.154607860978349,1.74894552961493,1.64289183246942));
#5606=CARTESIAN_POINT('Ctrl Pts',(0.198945932189457,1.70460745840382,1.63811406745469));
#5607=CARTESIAN_POINT('Ctrl Pts',(0.218177859368546,1.67652816181843,1.63556247215209));
#5608=CARTESIAN_POINT('Ctrl Pts',(0.243706194926033,1.61494799959182,1.63195388134767));
#5609=CARTESIAN_POINT('Ctrl Pts',(0.25,1.58144291640553,1.63095064303001));
#5610=CARTESIAN_POINT('Ctrl Pts',(0.25,1.51855708359447,1.63095064303001));
#5611=CARTESIAN_POINT('Ctrl Pts',(0.243706194926033,1.48505200040818,1.63195388134767));
#5612=CARTESIAN_POINT('Ctrl Pts',(0.218177859368546,1.42347183818157,1.63556247215209));
#5613=CARTESIAN_POINT('Ctrl Pts',(0.198945932189457,1.39539254159618,1.63811406745469));
#5614=CARTESIAN_POINT('Ctrl Pts',(0.154607860978348,1.35105447038507,1.64289183246942));
#5615=CARTESIAN_POINT('Ctrl Pts',(0.126528390765307,1.33182222741682,1.64543058688707));
#5616=CARTESIAN_POINT('Ctrl Pts',(0.0649476351123397,1.30629366210296,1.64900971937348));
#5617=CARTESIAN_POINT('Ctrl Pts',(0.0314423454288488,1.3,1.65));
#5618=CARTESIAN_POINT('Ctrl Pts',(-1.38777878078145E-17,1.3,1.65));
#5619=CARTESIAN_POINT('',(-0.25,1.55,1.63095064303001));
#5620=CARTESIAN_POINT('Ctrl Pts',(-5.55111512312578E-17,1.3,1.65));
#5621=CARTESIAN_POINT('Ctrl Pts',(-0.031442345428849,1.3,1.65));
#5622=CARTESIAN_POINT('Ctrl Pts',(-0.0649476351123398,1.30629366210296,
1.64900971937348));
#5623=CARTESIAN_POINT('Ctrl Pts',(-0.126528390765307,1.33182222741682,1.64543058688707));
#5624=CARTESIAN_POINT('Ctrl Pts',(-0.154607860978349,1.35105447038507,1.64289183246942));
#5625=CARTESIAN_POINT('Ctrl Pts',(-0.198945932189457,1.39539254159618,1.63811406745469));
#5626=CARTESIAN_POINT('Ctrl Pts',(-0.218177859368546,1.42347183818157,1.63556247215209));
#5627=CARTESIAN_POINT('Ctrl Pts',(-0.243706194926033,1.48505200040818,1.63195388134767));
#5628=CARTESIAN_POINT('Ctrl Pts',(-0.25,1.51855708359447,1.63095064303001));
#5629=CARTESIAN_POINT('Ctrl Pts',(-0.25,1.55,1.63095064303001));
#5630=CARTESIAN_POINT('Ctrl Pts',(-0.25,1.55,1.63095064303001));
#5631=CARTESIAN_POINT('Ctrl Pts',(-0.25,1.58144291640553,1.63095064303001));
#5632=CARTESIAN_POINT('Ctrl Pts',(-0.243706194926033,1.61494799959182,1.63195388134767));
#5633=CARTESIAN_POINT('Ctrl Pts',(-0.218177859368546,1.67652816181843,1.63556247215209));
#5634=CARTESIAN_POINT('Ctrl Pts',(-0.198945932189456,1.70460745840382,1.63811406745469));
#5635=CARTESIAN_POINT('Ctrl Pts',(-0.154607860978348,1.74894552961493,1.64289183246942));
#5636=CARTESIAN_POINT('Ctrl Pts',(-0.126528390765307,1.76817777258318,1.64543058688707));
#5637=CARTESIAN_POINT('Ctrl Pts',(-0.0649476351123396,1.79370633789704,
1.64900971937348));
#5638=CARTESIAN_POINT('Ctrl Pts',(-0.0314423454288488,1.8,1.65));
#5639=CARTESIAN_POINT('Ctrl Pts',(7.63278329429795E-17,1.8,1.65));
#5640=CARTESIAN_POINT('Origin',(0.,1.55,0.));
#5641=CARTESIAN_POINT('',(-0.34736109069228,1.55,0.489224153812002));
#5642=CARTESIAN_POINT('',(0.125,1.55,0.21650635094611));
#5643=CARTESIAN_POINT('Ctrl Pts',(-0.34736109069228,1.55,0.489224153812002));
#5644=CARTESIAN_POINT('Ctrl Pts',(-0.34736109069228,1.58183602855499,0.489224153812002));
#5645=CARTESIAN_POINT('Ctrl Pts',(-0.353251858758695,1.61548166177648,0.485186294875824));
#5646=CARTESIAN_POINT('Ctrl Pts',(-0.375307371004242,1.67693412158597,0.468334260082228));
#5647=CARTESIAN_POINT('Ctrl Pts',(-0.391292050254279,1.70478184753241,0.455434178332924));
#5648=CARTESIAN_POINT('Ctrl Pts',(-0.425012071836758,1.74874496453875,0.424138206994599));
#5649=CARTESIAN_POINT('Ctrl Pts',(-0.445091520936419,1.76792916820474,0.403563860606914));
#5650=CARTESIAN_POINT('Ctrl Pts',(-0.484488022261587,1.79356669468566,0.355304950761552));
#5651=CARTESIAN_POINT('Ctrl Pts',(-0.503716463284046,1.8,0.32753749298313));
#5652=CARTESIAN_POINT('Ctrl Pts',(-0.535514021257281,1.8,0.27246250701687));
#5653=CARTESIAN_POINT('Ctrl Pts',(-0.549947124580677,1.79356669468566,0.241926459727038));
#5654=CARTESIAN_POINT('Ctrl Pts',(-0.572042315803119,1.76792916820474,0.183678633836535));
#5655=CARTESIAN_POINT('Ctrl Pts',(-0.579820497891285,1.74874496453875,0.156002147628389));
#5656=CARTESIAN_POINT('Ctrl Pts',(-0.590063593315144,1.70478184753241,0.11115176665264));
#5657=CARTESIAN_POINT('Ctrl Pts',(-0.593243052195919,1.67693412158597,0.0908585874761102));
#5658=CARTESIAN_POINT('Ctrl Pts',(-0.596809586309859,1.61548166177648,0.0633319361811903));
#5659=CARTESIAN_POINT('Ctrl Pts',(-0.59736109069228,1.58183602855499,0.0562114519197831));
#5660=CARTESIAN_POINT('Ctrl Pts',(-0.59736109069228,1.51816397144501,0.0562114519197831));
#5661=CARTESIAN_POINT('Ctrl Pts',(-0.596809586309859,1.48451833822352,0.0633319361811902));
#5662=CARTESIAN_POINT('Ctrl Pts',(-0.593243052195919,1.42306587841403,0.0908585874761101));
#5663=CARTESIAN_POINT('Ctrl Pts',(-0.590063593315144,1.39521815246759,0.11115176665264));
#5664=CARTESIAN_POINT('Ctrl Pts',(-0.579820497891285,1.35125503546125,0.156002147628389));
#5665=CARTESIAN_POINT('Ctrl Pts',(-0.572042315803119,1.33207083179526,0.183678633836535));
#5666=CARTESIAN_POINT('Ctrl Pts',(-0.549947124580676,1.30643330531434,0.241926459727038));
#5667=CARTESIAN_POINT('Ctrl Pts',(-0.535514021257281,1.3,0.27246250701687));
#5668=CARTESIAN_POINT('Ctrl Pts',(-0.503716463284046,1.3,0.32753749298313));
#5669=CARTESIAN_POINT('Ctrl Pts',(-0.484488022261587,1.30643330531434,0.355304950761552));
#5670=CARTESIAN_POINT('Ctrl Pts',(-0.445091520936419,1.33207083179526,0.403563860606914));
#5671=CARTESIAN_POINT('Ctrl Pts',(-0.425012071836758,1.35125503546125,0.424138206994599));
#5672=CARTESIAN_POINT('Ctrl Pts',(-0.391292050254279,1.39521815246759,0.455434178332924));
#5673=CARTESIAN_POINT('Ctrl Pts',(-0.375307371004241,1.42306587841403,0.468334260082228));
#5674=CARTESIAN_POINT('Ctrl Pts',(-0.353251858758695,1.48451833822352,0.485186294875824));
#5675=CARTESIAN_POINT('Ctrl Pts',(-0.34736109069228,1.51816397144501,0.489224153812002));
#5676=CARTESIAN_POINT('Ctrl Pts',(-0.34736109069228,1.55,0.489224153812002));
#5677=CARTESIAN_POINT('Origin',(0.,1.55,0.));
#5678=CARTESIAN_POINT('',(0.59736109069228,1.55,-0.0562114519197831));
#5679=CARTESIAN_POINT('Ctrl Pts',(0.59736109069228,1.55,-0.0562114519197831));
#5680=CARTESIAN_POINT('Ctrl Pts',(0.59736109069228,1.51816397144501,-0.0562114519197831));
#5681=CARTESIAN_POINT('Ctrl Pts',(0.596809586309859,1.48451833822352,-0.0633319361811902));
#5682=CARTESIAN_POINT('Ctrl Pts',(0.593243052195919,1.42306587841403,-0.0908585874761101));
#5683=CARTESIAN_POINT('Ctrl Pts',(0.590063593315144,1.39521815246759,-0.11115176665264));
#5684=CARTESIAN_POINT('Ctrl Pts',(0.579820497891285,1.35125503546125,-0.156002147628389));
#5685=CARTESIAN_POINT('Ctrl Pts',(0.572042315803119,1.33207083179526,-0.183678633836535));
#5686=CARTESIAN_POINT('Ctrl Pts',(0.549947124580677,1.30643330531434,-0.241926459727038));
#5687=CARTESIAN_POINT('Ctrl Pts',(0.535514021257281,1.3,-0.27246250701687));
#5688=CARTESIAN_POINT('Ctrl Pts',(0.503716463284046,1.3,-0.32753749298313));
#5689=CARTESIAN_POINT('Ctrl Pts',(0.484488022261587,1.30643330531434,-0.355304950761552));
#5690=CARTESIAN_POINT('Ctrl Pts',(0.445091520936419,1.33207083179526,-0.403563860606914));
#5691=CARTESIAN_POINT('Ctrl Pts',(0.425012071836758,1.35125503546125,-0.424138206994599));
#5692=CARTESIAN_POINT('Ctrl Pts',(0.391292050254279,1.39521815246759,-0.455434178332924));
#5693=CARTESIAN_POINT('Ctrl Pts',(0.375307371004241,1.42306587841403,-0.468334260082228));
#5694=CARTESIAN_POINT('Ctrl Pts',(0.353251858758695,1.48451833822352,-0.485186294875824));
#5695=CARTESIAN_POINT('Ctrl Pts',(0.34736109069228,1.51816397144501,-0.489224153812002));
#5696=CARTESIAN_POINT('Ctrl Pts',(0.34736109069228,1.58183602855499,-0.489224153812002));
#5697=CARTESIAN_POINT('Ctrl Pts',(0.353251858758695,1.61548166177647,-0.485186294875824));
#5698=CARTESIAN_POINT('Ctrl Pts',(0.375307371004241,1.67693412158597,-0.468334260082228));
#5699=CARTESIAN_POINT('Ctrl Pts',(0.391292050254279,1.70478184753241,-0.455434178332924));
#5700=CARTESIAN_POINT('Ctrl Pts',(0.425012071836758,1.74874496453875,-0.424138206994599));
#5701=CARTESIAN_POINT('Ctrl Pts',(0.445091520936419,1.76792916820474,-0.403563860606914));
#5702=CARTESIAN_POINT('Ctrl Pts',(0.484488022261587,1.79356669468566,-0.355304950761552));
#5703=CARTESIAN_POINT('Ctrl Pts',(0.503716463284046,1.8,-0.32753749298313));
#5704=CARTESIAN_POINT('Ctrl Pts',(0.535514021257281,1.8,-0.27246250701687));
#5705=CARTESIAN_POINT('Ctrl Pts',(0.549947124580677,1.79356669468566,-0.241926459727038));
#5706=CARTESIAN_POINT('Ctrl Pts',(0.572042315803119,1.76792916820474,-0.183678633836535));
#5707=CARTESIAN_POINT('Ctrl Pts',(0.579820497891285,1.74874496453875,-0.156002147628389));
#5708=CARTESIAN_POINT('Ctrl Pts',(0.590063593315144,1.70478184753241,-0.111151766652641));
#5709=CARTESIAN_POINT('Ctrl Pts',(0.593243052195919,1.67693412158597,-0.0908585874761104));
#5710=CARTESIAN_POINT('Ctrl Pts',(0.596809586309859,1.61548166177648,-0.0633319361811903));
#5711=CARTESIAN_POINT('Ctrl Pts',(0.59736109069228,1.58183602855499,-0.0562114519197831));
#5712=CARTESIAN_POINT('Ctrl Pts',(0.59736109069228,1.55,-0.0562114519197831));
#5713=CARTESIAN_POINT('',(0.125,1.55,0.21650635094611));
#5714=CARTESIAN_POINT('Origin',(0.,1.55,0.));
#5715=CARTESIAN_POINT('',(-0.25,1.55,-0.545435605731786));
#5716=CARTESIAN_POINT('',(-0.25,1.55,0.));
#5717=CARTESIAN_POINT('Ctrl Pts',(-0.25,1.55,-0.545435605731786));
#5718=CARTESIAN_POINT('Ctrl Pts',(-0.25,1.58183602855499,-0.545435605731786));
#5719=CARTESIAN_POINT('Ctrl Pts',(-0.243557727551164,1.61548166177648,-0.548518231057014));
#5720=CARTESIAN_POINT('Ctrl Pts',(-0.217935681191677,1.67693412158597,-0.559192847558338));
#5721=CARTESIAN_POINT('Ctrl Pts',(-0.198771543060865,1.70478184753241,-0.566585944985565));
#5722=CARTESIAN_POINT('Ctrl Pts',(-0.154808426054527,1.74874496453875,-0.580140354622989));
#5723=CARTESIAN_POINT('Ctrl Pts',(-0.1269507948667,1.76792916820474,-0.587242494443449));
#5724=CARTESIAN_POINT('Ctrl Pts',(-0.0654591023190899,1.79356669468566,
-0.597231410488591));
#5725=CARTESIAN_POINT('Ctrl Pts',(-0.0317975579732349,1.8,-0.6));
#5726=CARTESIAN_POINT('Ctrl Pts',(0.0317975579732349,1.8,-0.6));
#5727=CARTESIAN_POINT('Ctrl Pts',(0.0654591023190898,1.79356669468566,-0.597231410488591));
#5728=CARTESIAN_POINT('Ctrl Pts',(0.1269507948667,1.76792916820474,-0.587242494443449));
#5729=CARTESIAN_POINT('Ctrl Pts',(0.154808426054527,1.74874496453875,-0.580140354622989));
#5730=CARTESIAN_POINT('Ctrl Pts',(0.198771543060865,1.70478184753241,-0.566585944985565));
#5731=CARTESIAN_POINT('Ctrl Pts',(0.217935681191677,1.67693412158597,-0.559192847558338));
#5732=CARTESIAN_POINT('Ctrl Pts',(0.243557727551164,1.61548166177648,-0.548518231057014));
#5733=CARTESIAN_POINT('Ctrl Pts',(0.25,1.58183602855499,-0.545435605731786));
#5734=CARTESIAN_POINT('Ctrl Pts',(0.25,1.51816397144501,-0.545435605731786));
#5735=CARTESIAN_POINT('Ctrl Pts',(0.243557727551164,1.48451833822352,-0.548518231057014));
#5736=CARTESIAN_POINT('Ctrl Pts',(0.217935681191677,1.42306587841403,-0.559192847558338));
#5737=CARTESIAN_POINT('Ctrl Pts',(0.198771543060865,1.39521815246759,-0.566585944985565));
#5738=CARTESIAN_POINT('Ctrl Pts',(0.154808426054527,1.35125503546125,-0.580140354622989));
#5739=CARTESIAN_POINT('Ctrl Pts',(0.1269507948667,1.33207083179526,-0.587242494443449));
#5740=CARTESIAN_POINT('Ctrl Pts',(0.0654591023190899,1.30643330531434,-0.597231410488591));
#5741=CARTESIAN_POINT('Ctrl Pts',(0.0317975579732349,1.3,-0.6));
#5742=CARTESIAN_POINT('Ctrl Pts',(-0.0317975579732349,1.3,-0.6));
#5743=CARTESIAN_POINT('Ctrl Pts',(-0.0654591023190899,1.30643330531434,
-0.597231410488591));
#5744=CARTESIAN_POINT('Ctrl Pts',(-0.1269507948667,1.33207083179526,-0.587242494443449));
#5745=CARTESIAN_POINT('Ctrl Pts',(-0.154808426054527,1.35125503546125,-0.580140354622989));
#5746=CARTESIAN_POINT('Ctrl Pts',(-0.198771543060865,1.39521815246759,-0.566585944985565));
#5747=CARTESIAN_POINT('Ctrl Pts',(-0.217935681191677,1.42306587841403,-0.559192847558338));
#5748=CARTESIAN_POINT('Ctrl Pts',(-0.243557727551164,1.48451833822352,-0.548518231057014));
#5749=CARTESIAN_POINT('Ctrl Pts',(-0.25,1.51816397144501,-0.545435605731786));
#5750=CARTESIAN_POINT('Ctrl Pts',(-0.25,1.55,-0.545435605731786));
#5751=CARTESIAN_POINT('Origin',(0.,1.55,0.));
#5752=CARTESIAN_POINT('',(-0.25,1.55,0.545435605731786));
#5753=CARTESIAN_POINT('Ctrl Pts',(-0.25,1.55,0.545435605731786));
#5754=CARTESIAN_POINT('Ctrl Pts',(-0.25,1.51816397144501,0.545435605731786));
#5755=CARTESIAN_POINT('Ctrl Pts',(-0.243557727551164,1.48451833822352,0.548518231057014));
#5756=CARTESIAN_POINT('Ctrl Pts',(-0.217935681191677,1.42306587841403,0.559192847558338));
#5757=CARTESIAN_POINT('Ctrl Pts',(-0.198771543060865,1.39521815246759,0.566585944985565));
#5758=CARTESIAN_POINT('Ctrl Pts',(-0.154808426054527,1.35125503546125,0.580140354622989));
#5759=CARTESIAN_POINT('Ctrl Pts',(-0.1269507948667,1.33207083179526,0.587242494443449));
#5760=CARTESIAN_POINT('Ctrl Pts',(-0.0654591023190899,1.30643330531434,
0.597231410488591));
#5761=CARTESIAN_POINT('Ctrl Pts',(-0.0317975579732349,1.3,0.6));
#5762=CARTESIAN_POINT('Ctrl Pts',(0.0317975579732349,1.3,0.6));
#5763=CARTESIAN_POINT('Ctrl Pts',(0.0654591023190899,1.30643330531434,0.597231410488591));
#5764=CARTESIAN_POINT('Ctrl Pts',(0.1269507948667,1.33207083179526,0.587242494443449));
#5765=CARTESIAN_POINT('Ctrl Pts',(0.154808426054527,1.35125503546125,0.580140354622989));
#5766=CARTESIAN_POINT('Ctrl Pts',(0.198771543060865,1.39521815246759,0.566585944985565));
#5767=CARTESIAN_POINT('Ctrl Pts',(0.217935681191677,1.42306587841403,0.559192847558338));
#5768=CARTESIAN_POINT('Ctrl Pts',(0.243557727551164,1.48451833822352,0.548518231057014));
#5769=CARTESIAN_POINT('Ctrl Pts',(0.25,1.51816397144501,0.545435605731786));
#5770=CARTESIAN_POINT('Ctrl Pts',(0.25,1.58183602855499,0.545435605731786));
#5771=CARTESIAN_POINT('Ctrl Pts',(0.243557727551164,1.61548166177648,0.548518231057014));
#5772=CARTESIAN_POINT('Ctrl Pts',(0.217935681191677,1.67693412158597,0.559192847558338));
#5773=CARTESIAN_POINT('Ctrl Pts',(0.198771543060865,1.70478184753241,0.566585944985565));
#5774=CARTESIAN_POINT('Ctrl Pts',(0.154808426054527,1.74874496453875,0.580140354622989));
#5775=CARTESIAN_POINT('Ctrl Pts',(0.1269507948667,1.76792916820474,0.587242494443449));
#5776=CARTESIAN_POINT('Ctrl Pts',(0.0654591023190898,1.79356669468566,0.597231410488591));
#5777=CARTESIAN_POINT('Ctrl Pts',(0.0317975579732349,1.8,0.6));
#5778=CARTESIAN_POINT('Ctrl Pts',(-0.0317975579732349,1.8,0.6));
#5779=CARTESIAN_POINT('Ctrl Pts',(-0.0654591023190898,1.79356669468566,
0.597231410488591));
#5780=CARTESIAN_POINT('Ctrl Pts',(-0.1269507948667,1.76792916820474,0.587242494443449));
#5781=CARTESIAN_POINT('Ctrl Pts',(-0.154808426054527,1.74874496453875,0.580140354622989));
#5782=CARTESIAN_POINT('Ctrl Pts',(-0.198771543060865,1.70478184753241,0.566585944985565));
#5783=CARTESIAN_POINT('Ctrl Pts',(-0.217935681191677,1.67693412158597,0.559192847558339));
#5784=CARTESIAN_POINT('Ctrl Pts',(-0.243557727551164,1.61548166177648,0.548518231057014));
#5785=CARTESIAN_POINT('Ctrl Pts',(-0.25,1.58183602855499,0.545435605731786));
#5786=CARTESIAN_POINT('Ctrl Pts',(-0.25,1.55,0.545435605731786));
#5787=CARTESIAN_POINT('',(-0.25,1.55,0.));
#5788=CARTESIAN_POINT('Origin',(1.65,2.25,0.));
#5789=CARTESIAN_POINT('',(-0.6,2.25,-7.34788079488412E-17));
#5790=CARTESIAN_POINT('Origin',(0.,2.25,0.));
#5791=CARTESIAN_POINT('Origin',(1.75,0.85,0.));
#5792=CARTESIAN_POINT('',(-1.75,0.85,-2.14313189850787E-16));
#5793=CARTESIAN_POINT('Origin',(0.,0.85,0.));
#5794=CARTESIAN_POINT('Origin',(0.,0.,0.));
#5795=CARTESIAN_POINT('',(-1.75,-0.85,-2.14313189850787E-16));
#5796=CARTESIAN_POINT('Origin',(0.,-0.85,0.));
#5797=CARTESIAN_POINT('',(-1.75,0.,-2.14313189850787E-16));
#5798=CARTESIAN_POINT('Origin',(0.6,-0.85,0.));
#5799=CARTESIAN_POINT('',(-0.6,-0.85,-7.34788079488412E-17));
#5800=CARTESIAN_POINT('Origin',(0.,-0.85,0.));
#5801=CARTESIAN_POINT('Origin',(0.,0.7,0.));
#5802=CARTESIAN_POINT('',(-0.6,0.7,-7.34788079488412E-17));
#6769=UNCERTAINTY_MEASURE_WITH_UNIT(LENGTH_MEASURE(0.001),#6806,
'DISTANCE_ACCURACY_VALUE',
'Maximum model space distance between geometric entities at asserted c
onnectivities');
#6780=UNCERTAINTY_MEASURE_WITH_UNIT(LENGTH_MEASURE(0.001),#6806,
'DISTANCE_ACCURACY_VALUE',
'Maximum model space distance between geometric entities at asserted c
onnectivities');
#6794=(
GEOMETRIC_REPRESENTATION_CONTEXT(3)
GLOBAL_UNCERTAINTY_ASSIGNED_CONTEXT((#6769))
GLOBAL_UNIT_ASSIGNED_CONTEXT((#6806,#6808,#6809))
REPRESENTATION_CONTEXT('','3D')
);
#6805=(
GEOMETRIC_REPRESENTATION_CONTEXT(3)
GLOBAL_UNCERTAINTY_ASSIGNED_CONTEXT((#6780))
GLOBAL_UNIT_ASSIGNED_CONTEXT((#6806,#6808,#6809))
REPRESENTATION_CONTEXT('','3D')
);
#6806=(
LENGTH_UNIT()
NAMED_UNIT(*)
SI_UNIT(.CENTI.,.METRE.)
);
#6808=(
NAMED_UNIT(*)
PLANE_ANGLE_UNIT()
SI_UNIT($,.RADIAN.)
);
#6809=(
NAMED_UNIT(*)
SI_UNIT($,.STERADIAN.)
SOLID_ANGLE_UNIT()
);
#6823=SHAPE_DEFINITION_REPRESENTATION(#6847,#6911);
#6847=PRODUCT_DEFINITION_SHAPE('',$,#6936);
#6911=SHAPE_REPRESENTATION('',(#3713),#6794);
#6922=PRODUCT_DEFINITION_CONTEXT('part definition',#6996,'design');
#6936=PRODUCT_DEFINITION('Insert bearing','Insert bearing',#6960,#6922);
#6960=PRODUCT_DEFINITION_FORMATION('',$,#7011);
#6996=APPLICATION_CONTEXT(
'Core Data for Automotive Mechanical Design Process');
#6997=PRODUCT_CONTEXT('part definition',#6996,'mechanical');
#7011=PRODUCT('Insert bearing','Insert bearing','Insert bearing',(#6997));
#7085=COLOUR_RGB('Grey',0.48,0.52,0.57);
#7086=FILL_AREA_STYLE_COLOUR('',#7085);
#7087=FILL_AREA_STYLE('',(#7086));
#7088=SURFACE_STYLE_FILL_AREA(#7087);
#7089=SURFACE_SIDE_STYLE('',(#7088));
#7090=SURFACE_STYLE_USAGE(.BOTH.,#7089);
#7091=PRESENTATION_STYLE_ASSIGNMENT((#7090));
ENDSEC;
END-ISO-10303-21;
